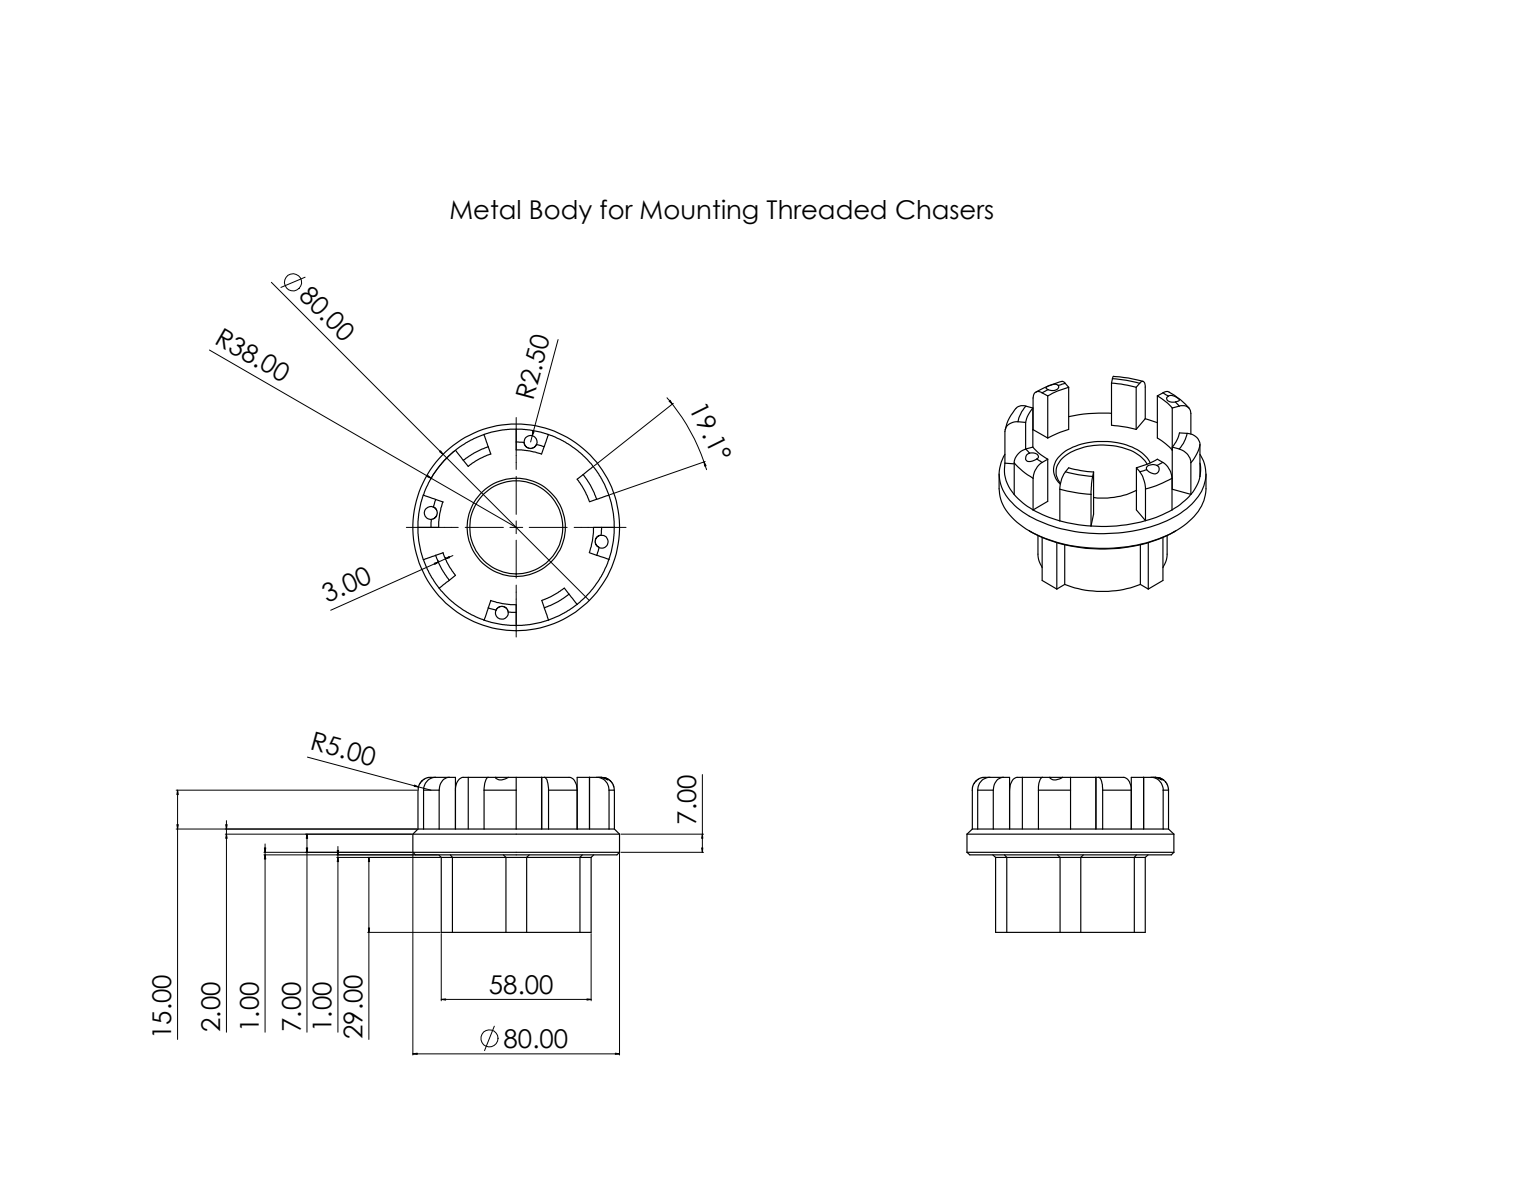
ISO-10303-21;
HEADER;
FILE_DESCRIPTION (('STEP AP214'),
    '1' );
FILE_NAME ('Metal Body for Mounting Threaded Chasers.step',
    '2026-10-19T14:05:14',
    ( '' ),
    ( '' ),
    'SwSTEP 2.0',
    'SolidWorks 2025',
    '' );
FILE_SCHEMA (( 'AUTOMOTIVE_DESIGN' ));
ENDSEC;

DATA;
#1=AXIS2_PLACEMENT_3D ( 'NONE', #3987, #6980, #243 ) ;
#2=CARTESIAN_POINT ( 'NONE',  ( -12.48950176432141923, 54.99999999999999289, -35.88888888888889284 ) ) ;
#16=CARTESIAN_POINT ( 'NONE',  ( 0.000000000000000000, 39.99999999999999289, 0.000000000000000000 ) ) ;
#17=ORIENTED_EDGE ( 'NONE', *, *, #1471, .T. ) ;
#22=VERTEX_POINT ( 'NONE', #2863 ) ;
#23=CARTESIAN_POINT ( 'NONE',  ( -7.995545880304240960, 59.98659813632739457, 32.45264704635820152 ) ) ;
#26=ORIENTED_EDGE ( 'NONE', *, *, #454, .F. ) ;
#28=AXIS2_PLACEMENT_3D ( 'NONE', #4537, #730, #2939 ) ;
#31=DIRECTION ( 'NONE',  ( 0.000000000000000000, 0.000000000000000000, 1.000000000000000000 ) ) ;
#33=CARTESIAN_POINT ( 'NONE',  ( 28.34870838944214100, 59.99999999999999289, 9.815840903884559765 ) ) ;
#39=VECTOR ( 'NONE', #8891, 1000.000000000000000 ) ;
#40=CARTESIAN_POINT ( 'NONE',  ( -8.673617379884032514E-16, 30.00000000000000000, -4.000000000000002665 ) ) ;
#48=ADVANCED_FACE ( 'NONE', ( #1481 ), #9105, .T. ) ;
#52=ORIENTED_EDGE ( 'NONE', *, *, #3525, .F. ) ;
#53=CARTESIAN_POINT ( 'NONE',  ( 38.00000000000000711, 59.99999999999999289, 1.288922537256478387E-13 ) ) ;
#59=DIRECTION ( 'NONE',  ( -1.000000000000000000, 0.000000000000000000, 1.084202172485503448E-16 ) ) ;
#60=ORIENTED_EDGE ( 'NONE', *, *, #1877, .F. ) ;
#61=AXIS2_PLACEMENT_3D ( 'NONE', #6025, #2270, #8317 ) ;
#63=PRODUCT_CONTEXT ( 'NONE', #3923, 'mechanical' ) ;
#68=CARTESIAN_POINT ( 'NONE',  ( -3.999999999999999112, 28.99999999999997158, 24.67792535850613334 ) ) ;
#69=ORIENTED_EDGE ( 'NONE', *, *, #3277, .T. ) ;
#71=VERTEX_POINT ( 'NONE', #9199 ) ;
#73=DIRECTION ( 'NONE',  ( 0.000000000000000000, 1.000000000000000000, 0.000000000000000000 ) ) ;
#74=EDGE_CURVE ( 'NONE', #2204, #4788, #7083, .T. ) ;
#78=CARTESIAN_POINT ( 'NONE',  ( 28.33333333333337478, 39.99999999999999289, -9.860132971832594961 ) ) ;
#79=CARTESIAN_POINT ( 'NONE',  ( 20.99999999999999645, 30.00000000000000000, 4.000000000000000888 ) ) ;
#86=DIRECTION ( 'NONE',  ( 0.000000000000000000, 0.000000000000000000, 1.000000000000000000 ) ) ;
#91=ORIENTED_EDGE ( 'NONE', *, *, #7636, .T. ) ;
#92=CARTESIAN_POINT ( 'NONE',  ( 5.562309845534588959, 49.99999999999999289, -33.06426808735054124 ) ) ;
#95=CARTESIAN_POINT ( 'NONE',  ( 24.67792535850613334, 0.000000000000000000, 4.000000000000000888 ) ) ;
#96=CARTESIAN_POINT ( 'NONE',  ( 0.000000000000000000, 0.000000000000000000, 0.000000000000000000 ) ) ;
#99=DIRECTION ( 'NONE',  ( 0.9449569463147374782, 0.000000000000000000, 0.3271946967961527619 ) ) ;
#101=DIRECTION ( 'NONE',  ( 0.000000000000000000, -1.000000000000000000, 0.000000000000000000 ) ) ;
#105=AXIS2_PLACEMENT_3D ( 'NONE', #139, #1748, #4771 ) ;
#106=EDGE_CURVE ( 'NONE', #1933, #8061, #806, .T. ) ;
#108=VECTOR ( 'NONE', #4796, 1000.000000000000000 ) ;
#115=ADVANCED_FACE ( 'NONE', ( #5243 ), #6016, .F. ) ;
#120=CLOSED_SHELL ( 'NONE', ( #1419, #7952, #2099, #3958, #3679, #8907, #3700, #3725, #1256, #288, #9736, #7646, #7332, #6776, #8180, #48, #7507, #2171, #4864, #7401, #2702, #2733, #7456, #636, #936, #1118, #6024, #1058, #540, #1404, #1588, #7209, #115, #1059, #588, #939, #8009, #6508, #1237, #2007, #4157, #6912, #2948, #702, #4090, #7822, #4876, #3409, #2741, #2560, #1004, #4751, #8856, #1093, #818, #5216, #1926, #9214, #9112, #7707, #4600, #634, #1660, #1234, #9684, #1433, #2142, #7068, #5305, #2300, #8588, #5110, #8978, #5514, #6739, #8244, #7533, #7708, #9094, #6502, #6348, #7871, #6449, #6840, #9282, #4029, #5531, #4774, #891, #5599, #3099, #5594, #5412, #1186, #7274, #6763, #3544, #3838, #1663, #3596, #7633, #5416, #9580, #6826, #5045, #4533, #1363 ) ) ;
#121=ORIENTED_EDGE ( 'NONE', *, *, #2139, .T. ) ;
#123=ORIENTED_EDGE ( 'NONE', *, *, #454, .T. ) ;
#127=LINE ( 'NONE', #9051, #3388 ) ;
#130=ORIENTED_EDGE ( 'NONE', *, *, #5654, .T. ) ;
#132=CARTESIAN_POINT ( 'NONE',  ( 4.000000000000001776, 28.99999999999997158, -24.67792535850613334 ) ) ;
#135=DIRECTION ( 'NONE',  ( -0.000000000000000000, -1.000000000000000000, -0.000000000000000000 ) ) ;
#137=VERTEX_POINT ( 'NONE', #6145 ) ;
#139=CARTESIAN_POINT ( 'NONE',  ( 0.000000000000000000, 54.99999999999999289, 0.000000000000000000 ) ) ;
#140=CARTESIAN_POINT ( 'NONE',  ( 32.85680095556730862, 59.99999999999999289, 3.070933240276029874 ) ) ;
#141=ORIENTED_EDGE ( 'NONE', *, *, #4576, .F. ) ;
#142=DIRECTION ( 'NONE',  ( -0.000000000000000000, -1.000000000000000000, -0.000000000000000000 ) ) ;
#143=ORIENTED_EDGE ( 'NONE', *, *, #5654, .F. ) ;
#151=CARTESIAN_POINT ( 'NONE',  ( 4.000000000000007994, 30.00000000000000000, 24.67792535850613334 ) ) ;
#152=CARTESIAN_POINT ( 'NONE',  ( 5.562309845534588959, 59.99999999999999289, -30.56426808735054479 ) ) ;
#156=VERTEX_POINT ( 'NONE', #6690 ) ;
#165=CARTESIAN_POINT ( 'NONE',  ( -4.331874290630486790, 29.33187429063046991, 24.96033808169876878 ) ) ;
#167=VERTEX_POINT ( 'NONE', #7496 ) ;
#174=CARTESIAN_POINT ( 'NONE',  ( 4.000000000000002665, 30.00000000000000000, -8.673617379884032514E-16 ) ) ;
#177=ORIENTED_EDGE ( 'NONE', *, *, #6292, .F. ) ;
#178=CARTESIAN_POINT ( 'NONE',  ( -7.935670091272695181, 60.00000000000000711, 32.24976038726180860 ) ) ;
#179=VERTEX_POINT ( 'NONE', #3191 ) ;
#183=CIRCLE ( 'NONE', #5688, 37.99999999999999289 ) ;
#186=CARTESIAN_POINT ( 'NONE',  ( -29.00000000000000355, 30.00000000000000000, 4.000000000000010658 ) ) ;
#187=LINE ( 'NONE', #9125, #4256 ) ;
#190=DIRECTION ( 'NONE',  ( 0.000000000000000000, -0.000000000000000000, 1.000000000000000000 ) ) ;
#191=CARTESIAN_POINT ( 'NONE',  ( 7.856683717344210116, 59.59863544270934455, -34.07748394475226661 ) ) ;
#192=LINE ( 'NONE', #2440, #6007 ) ;
#194=CARTESIAN_POINT ( 'NONE',  ( 0.000000000000000000, 54.99999999999999289, 0.000000000000000000 ) ) ;
#196=CARTESIAN_POINT ( 'NONE',  ( 12.43339847825378364, 39.99999999999999289, -35.90836395996003461 ) ) ;
#201=EDGE_CURVE ( 'NONE', #5205, #8953, #1759, .T. ) ;
#204=CARTESIAN_POINT ( 'NONE',  ( 33.06426808735054124, 59.99576382555915899, 3.062309845534584074 ) ) ;
#206=AXIS2_PLACEMENT_3D ( 'NONE', #7812, #2466, #1194 ) ;
#207=CARTESIAN_POINT ( 'NONE',  ( 0.000000000000000000, 30.00000000000000000, 0.000000000000000000 ) ) ;
#208=DIRECTION ( 'NONE',  ( 0.000000000000000000, -1.000000000000000000, 0.000000000000000000 ) ) ;
#209=VERTEX_POINT ( 'NONE', #7698 ) ;
#215=ORIENTED_EDGE ( 'NONE', *, *, #2320, .T. ) ;
#218=ORIENTED_EDGE ( 'NONE', *, *, #4973, .T. ) ;
#219=CARTESIAN_POINT ( 'NONE',  ( 33.06426808735054124, 49.99999999999999289, 5.562309845534586294 ) ) ;
#220=AXIS2_PLACEMENT_3D ( 'NONE', #9694, #2922, #5107 ) ;
#223=EDGE_CURVE ( 'NONE', #5194, #1935, #3139, .T. ) ;
#227=ORIENTED_EDGE ( 'NONE', *, *, #8008, .F. ) ;
#228=CARTESIAN_POINT ( 'NONE',  ( -33.72085295419949347, 59.72647237447257851, -7.995677060003914427 ) ) ;
#230=ORIENTED_EDGE ( 'NONE', *, *, #1372, .F. ) ;
#231=ORIENTED_EDGE ( 'NONE', *, *, #8364, .T. ) ;
#234=FACE_OUTER_BOUND ( 'NONE', #8971, .T. ) ;
#236=ORIENTED_EDGE ( 'NONE', *, *, #3146, .F. ) ;
#237=EDGE_CURVE ( 'NONE', #1437, #3718, #3681, .T. ) ;
#238=ORIENTED_EDGE ( 'NONE', *, *, #9403, .F. ) ;
#243=DIRECTION ( 'NONE',  ( 0.000000000000000000, 0.000000000000000000, 1.000000000000000000 ) ) ;
#247=ORIENTED_EDGE ( 'NONE', *, *, #9110, .F. ) ;
#252=VERTEX_POINT ( 'NONE', #7632 ) ;
#264=VECTOR ( 'NONE', #8760, 1000.000000000000000 ) ;
#267=CARTESIAN_POINT ( 'NONE',  ( 0.000000000000000000, 37.99999999999996447, -40.00000000000000711 ) ) ;
#268=PLANE ( 'NONE',  #1365 ) ;
#270=AXIS2_PLACEMENT_3D ( 'NONE', #2075, #7132, #3665 ) ;
#275=ORIENTED_EDGE ( 'NONE', *, *, #6897, .F. ) ;
#276=CARTESIAN_POINT ( 'NONE',  ( -35.47893788052810038, 58.98370868798952671, -6.231324730575372506 ) ) ;
#279=VERTEX_POINT ( 'NONE', #6422 ) ;
#280=EDGE_CURVE ( 'NONE', #8145, #2204, #7893, .T. ) ;
#287=CARTESIAN_POINT ( 'NONE',  ( 3.060768115627997776, 59.99034304420147379, -33.21665709534246957 ) ) ;
#288=ADVANCED_FACE ( 'NONE', ( #6098 ), #6191, .T. ) ;
#289=PLANE ( 'NONE',  #8040 ) ;
#290=EDGE_CURVE ( 'NONE', #22, #2244, #187, .T. ) ;
#291=CARTESIAN_POINT ( 'NONE',  ( 33.00000000000000711, 59.99999999999999289, 1.152188841818234386E-13 ) ) ;
#294=VERTEX_POINT ( 'NONE', #8424 ) ;
#295=CARTESIAN_POINT ( 'NONE',  ( -2.653525817520781855E-13, 39.99999999999999289, 38.00000000000000711 ) ) ;
#300=VERTEX_POINT ( 'NONE', #423 ) ;
#303=CARTESIAN_POINT ( 'NONE',  ( 0.000000000000000000, 28.99999999999997158, 0.000000000000000000 ) ) ;
#307=LINE ( 'NONE', #9387, #9703 ) ;
#308=ORIENTED_EDGE ( 'NONE', *, *, #4770, .F. ) ;
#310=ORIENTED_EDGE ( 'NONE', *, *, #635, .T. ) ;
#311=VECTOR ( 'NONE', #5751, 1000.000000000000000 ) ;
#312=DIRECTION ( 'NONE',  ( 0.000000000000000000, 1.000000000000000000, 0.000000000000000000 ) ) ;
#313=CARTESIAN_POINT ( 'NONE',  ( -5.562309845534584518, 49.99999999999999289, 35.56426808735054834 ) ) ;
#314=ORIENTED_EDGE ( 'NONE', *, *, #2672, .F. ) ;
#316=ORIENTED_EDGE ( 'NONE', *, *, #2562, .T. ) ;
#317=CARTESIAN_POINT ( 'NONE',  ( 0.000000000000000000, 1.000000000000014655, 0.000000000000000000 ) ) ;
#323=CARTESIAN_POINT ( 'NONE',  ( 23.54469556655648077, 59.99999999999999289, 29.82695610816123022 ) ) ;
#325=CIRCLE ( 'NONE', #6298, 38.00000000000000711 ) ;
#327=CARTESIAN_POINT ( 'NONE',  ( 2.326828918379978070E-15, 39.99999999999999289, -19.00000000000005684 ) ) ;
#330=DIRECTION ( 'NONE',  ( -0.9444444444444315412, 0.000000000000000000, 0.3286710990611268479 ) ) ;
#333=AXIS2_PLACEMENT_3D ( 'NONE', #8336, #1619, #1570 ) ;
#334=CARTESIAN_POINT ( 'NONE',  ( 33.06426808735054124, 49.99999999999999289, 3.062309845534584074 ) ) ;
#337=EDGE_CURVE ( 'NONE', #8698, #5898, #9303, .T. ) ;
#338=EDGE_LOOP ( 'NONE', ( #2836, #3852, #9165, #3920 ) ) ;
#339=CARTESIAN_POINT ( 'NONE',  ( -27.66666666666669272, 27.66666666666662167, 2.666666666666698049 ) ) ;
#342=DIRECTION ( 'NONE',  ( 0.000000000000000000, 0.000000000000000000, 1.000000000000000000 ) ) ;
#343=CARTESIAN_POINT ( 'NONE',  ( 0.000000000000000000, 0.000000000000000000, -19.00000000000000355 ) ) ;
#352=EDGE_CURVE ( 'NONE', #8330, #6149, #3299, .T. ) ;
#354=EDGE_LOOP ( 'NONE', ( #1511, #1589, #3120, #2364 ) ) ;
#355=DIRECTION ( 'NONE',  ( 0.000000000000000000, 0.000000000000000000, 1.000000000000000000 ) ) ;
#360=LINE ( 'NONE', #5642, #2706 ) ;
#361=CYLINDRICAL_SURFACE ( 'NONE', #4515, 2.500000000000002220 ) ;
#365=CARTESIAN_POINT ( 'NONE',  ( 4.000000000000001776, 28.99999999999997158, -29.00000000000000355 ) ) ;
#367=ORIENTED_EDGE ( 'NONE', *, *, #5413, .T. ) ;
#370=ORIENTED_EDGE ( 'NONE', *, *, #6332, .F. ) ;
#374=VECTOR ( 'NONE', #842, 1000.000000000000000 ) ;
#378=CARTESIAN_POINT ( 'NONE',  ( 29.00000000000000355, 0.000000000000000000, 4.000000000000000000 ) ) ;
#380=PLANE ( 'NONE',  #9644 ) ;
#381=LINE ( 'NONE', #8854, #6240 ) ;
#384=LINE ( 'NONE', #5665, #2838 ) ;
#389=CARTESIAN_POINT ( 'NONE',  ( 29.00000000000000355, 28.99999999999997158, 4.000000000000000000 ) ) ;
#394=ORIENTED_EDGE ( 'NONE', *, *, #7055, .T. ) ;
#396=EDGE_CURVE ( 'NONE', #1074, #9346, #9245, .T. ) ;
#397=CARTESIAN_POINT ( 'NONE',  ( -9.860132971832692661, 59.99999999999999289, -28.33333333333334281 ) ) ;
#401=DIRECTION ( 'NONE',  ( 0.000000000000000000, 0.000000000000000000, -1.000000000000000000 ) ) ;
#403=CARTESIAN_POINT ( 'NONE',  ( -25.51470164434615029, 30.00000000000000000, 5.000000000000010658 ) ) ;
#404=VECTOR ( 'NONE', #5914, 1000.000000000000000 ) ;
#405=CIRCLE ( 'NONE', #6383, 25.00000000000000000 ) ;
#406=ORIENTED_EDGE ( 'NONE', *, *, #5172, .F. ) ;
#407=CARTESIAN_POINT ( 'NONE',  ( 32.89361530837994962, 59.92713194881500982, 8.062309845534587183 ) ) ;
#410=ORIENTED_EDGE ( 'NONE', *, *, #3584, .F. ) ;
#413=CARTESIAN_POINT ( 'NONE',  ( -9.860132971832692661, 39.99999999999999289, -28.33333333333334281 ) ) ;
#418=AXIS2_PLACEMENT_3D ( 'NONE', #5812, #3538, #4432 ) ;
#423=CARTESIAN_POINT ( 'NONE',  ( -3.999999999999998224, 0.000000000000000000, 29.00000000000000355 ) ) ;
#427=VERTEX_POINT ( 'NONE', #5125 ) ;
#428=DIRECTION ( 'NONE',  ( 0.000000000000000000, 0.000000000000000000, 1.000000000000000000 ) ) ;
#430=ORIENTED_EDGE ( 'NONE', *, *, #1372, .T. ) ;
#437=ORIENTED_EDGE ( 'NONE', *, *, #7689, .F. ) ;
#438=FACE_OUTER_BOUND ( 'NONE', #6312, .T. ) ;
#439=FACE_OUTER_BOUND ( 'NONE', #470, .T. ) ;
#441=DIRECTION ( 'NONE',  ( 0.000000000000000000, 0.000000000000000000, 1.000000000000000000 ) ) ;
#446=ORIENTED_EDGE ( 'NONE', *, *, #6627, .T. ) ;
#448=DIRECTION ( 'NONE',  ( 0.000000000000000000, 0.7071067811865474617, 0.7071067811865474617 ) ) ;
#450=DIRECTION ( 'NONE',  ( 0.000000000000000000, 0.000000000000000000, 1.000000000000000000 ) ) ;
#452=DIRECTION ( 'NONE',  ( 0.7071067811865573427, -0.7071067811865376918, -0.000000000000000000 ) ) ;
#454=EDGE_CURVE ( 'NONE', #4849, #1467, #8923, .T. ) ;
#460=DIRECTION ( 'NONE',  ( 0.6195972517514876099, -0.000000000000000000, 0.7849198975831889191 ) ) ;
#470=EDGE_LOOP ( 'NONE', ( #5916, #4580, #3218, #2134, #8926 ) ) ;
#471=DIRECTION ( 'NONE',  ( 0.9444444444444359821, 0.000000000000000000, -0.3286710990611142469 ) ) ;
#472=EDGE_LOOP ( 'NONE', ( #7982, #7930, #8063, #3856 ) ) ;
#475=DIRECTION ( 'NONE',  ( -0.000000000000000000, -1.000000000000000000, -0.000000000000000000 ) ) ;
#479=DIRECTION ( 'NONE',  ( 0.000000000000000000, 0.000000000000000000, 1.000000000000000000 ) ) ;
#489=ORIENTED_EDGE ( 'NONE', *, *, #3270, .T. ) ;
#494=EDGE_LOOP ( 'NONE', ( #6497, #4079, #9500, #4446, #1743, #1658, #5716 ) ) ;
#504=VERTEX_POINT ( 'NONE', #5174 ) ;
#509=EDGE_CURVE ( 'NONE', #4792, #7168, #1410, .T. ) ;
#511=CIRCLE ( 'NONE', #8869, 5.000000000000001776 ) ;
#514=CARTESIAN_POINT ( 'NONE',  ( 0.000000000000000000, 30.00000000000000000, 0.000000000000000000 ) ) ;
#516=CARTESIAN_POINT ( 'NONE',  ( -4.000000000000005329, 28.99999999999997158, -29.00000000000000355 ) ) ;
#522=DIRECTION ( 'NONE',  ( -0.7849198975831889191, -0.000000000000000000, 0.6195972517514874989 ) ) ;
#527=ORIENTED_EDGE ( 'NONE', *, *, #2371, .T. ) ;
#529=CARTESIAN_POINT ( 'NONE',  ( 28.33333333333337833, 59.99999999999999289, -9.860132971832594961 ) ) ;
#531=CARTESIAN_POINT ( 'NONE',  ( 4.000000000000001776, 0.000000000000000000, 0.000000000000000000 ) ) ;
#533=VECTOR ( 'NONE', #5958, 1000.000000000000000 ) ;
#535=EDGE_CURVE ( 'NONE', #4621, #5147, #2943, .T. ) ;
#538=EDGE_CURVE ( 'NONE', #6765, #4792, #5901, .T. ) ;
#540=ADVANCED_FACE ( 'NONE', ( #4241, #5074 ), #1370, .F. ) ;
#542=AXIS2_PLACEMENT_3D ( 'NONE', #8748, #5544, #7870 ) ;
#547=FACE_OUTER_BOUND ( 'NONE', #7373, .T. ) ;
#551=SHAPE_REPRESENTATION ( 'Metal Body for Mounting Threaded Chasers', ( #6314 ), #2843 ) ;
#555=DIRECTION ( 'NONE',  ( -0.000000000000000000, -1.000000000000000000, -0.000000000000000000 ) ) ;
#557=ORIENTED_EDGE ( 'NONE', *, *, #2320, .F. ) ;
#558=DIRECTION ( 'NONE',  ( -0.000000000000000000, -1.000000000000000000, -0.000000000000000000 ) ) ;
#563=CARTESIAN_POINT ( 'NONE',  ( -34.19425402209839859, 59.81545713833158828, -3.326151553796970806 ) ) ;
#564=ORIENTED_EDGE ( 'NONE', *, *, #4438, .T. ) ;
#565=CARTESIAN_POINT ( 'NONE',  ( 33.72911585420148128, 59.92558239856793278, 3.146586008005429314 ) ) ;
#566=ORIENTED_EDGE ( 'NONE', *, *, #352, .T. ) ;
#568=ORIENTED_EDGE ( 'NONE', *, *, #7347, .T. ) ;
#573=AXIS2_PLACEMENT_3D ( 'NONE', #9355, #2572, #5602 ) ;
#575=DIRECTION ( 'NONE',  ( 0.000000000000000000, -0.7071067811865500152, -0.7071067811865451302 ) ) ;
#579=ORIENTED_EDGE ( 'NONE', *, *, #6665, .T. ) ;
#585=CARTESIAN_POINT ( 'NONE',  ( 4.331874290630496560, 29.33187429063046991, 24.96033808169876878 ) ) ;
#588=ADVANCED_FACE ( 'NONE', ( #8138 ), #2885, .T. ) ;
#590=DIRECTION ( 'NONE',  ( -1.000000000000000000, 0.000000000000000000, 2.168404344971006649E-16 ) ) ;
#592=EDGE_CURVE ( 'NONE', #7004, #2792, #2691, .T. ) ;
#593=ORIENTED_EDGE ( 'NONE', *, *, #4388, .T. ) ;
#595=DIRECTION ( 'NONE',  ( 0.000000000000000000, 1.000000000000000000, 0.000000000000000000 ) ) ;
#596=DIRECTION ( 'NONE',  ( -0.000000000000000000, -1.000000000000000000, -0.000000000000000000 ) ) ;
#598=ORIENTED_EDGE ( 'NONE', *, *, #5533, .T. ) ;
#602=CARTESIAN_POINT ( 'NONE',  ( -9.860132971832692661, 59.99999999999999289, -28.33333333333334281 ) ) ;
#604=EDGE_LOOP ( 'NONE', ( #4455, #8847, #6470, #2076 ) ) ;
#609=ORIENTED_EDGE ( 'NONE', *, *, #1964, .F. ) ;
#619=ORIENTED_EDGE ( 'NONE', *, *, #8790, .F. ) ;
#620=FACE_OUTER_BOUND ( 'NONE', #3521, .T. ) ;
#621=DIRECTION ( 'NONE',  ( 0.000000000000000000, -1.000000000000000000, 0.000000000000000000 ) ) ;
#622=DIRECTION ( 'NONE',  ( 0.000000000000000000, 0.000000000000000000, 1.000000000000000000 ) ) ;
#623=DIRECTION ( 'NONE',  ( 0.3271946967961529840, 0.000000000000000000, -0.9449569463147373671 ) ) ;
#624=DIRECTION ( 'NONE',  ( -0.000000000000000000, -1.000000000000000000, -0.000000000000000000 ) ) ;
#634=ADVANCED_FACE ( 'NONE', ( #4391 ), #5023, .F. ) ;
#635=EDGE_CURVE ( 'NONE', #5898, #2818, #5499, .T. ) ;
#636=ADVANCED_FACE ( 'NONE', ( #9571 ), #1321, .T. ) ;
#645=AXIS2_PLACEMENT_3D ( 'NONE', #194, #4729, #6198 ) ;
#654=ORIENTED_EDGE ( 'NONE', *, *, #4759, .F. ) ;
#655=DIRECTION ( 'NONE',  ( 0.000000000000000000, 0.000000000000000000, 1.000000000000000000 ) ) ;
#657=CARTESIAN_POINT ( 'NONE',  ( 35.48172963891341425, 59.13032414405947179, 4.904055200121585578 ) ) ;
#662=DIRECTION ( 'NONE',  ( 0.000000000000000000, 1.000000000000000000, 0.000000000000000000 ) ) ;
#666=ORIENTED_EDGE ( 'NONE', *, *, #2923, .F. ) ;
#674=CARTESIAN_POINT ( 'NONE',  ( 0.000000000000000000, 54.99999999999999289, 0.000000000000000000 ) ) ;
#685=B_SPLINE_CURVE_WITH_KNOTS ( 'NONE', 3,
 ( #9148, #1636, #3056, #5346 ),
 .UNSPECIFIED., .F., .F.,
 ( 4, 4 ),
 ( 0.000000000000000000, 0.001643226871903046308 ),
 .UNSPECIFIED. ) ;
#687=CARTESIAN_POINT ( 'NONE',  ( 20.99999999999999645, 30.00000000000000000, -4.000000000000006217 ) ) ;
#688=EDGE_LOOP ( 'NONE', ( #2555, #5795, #446, #121 ) ) ;
#690=EDGE_CURVE ( 'NONE', #5689, #4621, #1513, .T. ) ;
#691=ORIENTED_EDGE ( 'NONE', *, *, #2255, .T. ) ;
#697=LINE ( 'NONE', #6703, #2761 ) ;
#702=ADVANCED_FACE ( 'NONE', ( #881 ), #5993, .F. ) ;
#704=CARTESIAN_POINT ( 'NONE',  ( 35.54672840350796292, 58.97502204235875922, 5.902312647278757929 ) ) ;
#711=EDGE_LOOP ( 'NONE', ( #4221, #2161, #4934, #4957, #6130 ) ) ;
#712=DIRECTION ( 'NONE',  ( -0.000000000000000000, -1.000000000000000000, -0.000000000000000000 ) ) ;
#715=VECTOR ( 'NONE', #596, 1000.000000000000000 ) ;
#716=ORIENTED_EDGE ( 'NONE', *, *, #8054, .F. ) ;
#717=DIRECTION ( 'NONE',  ( 0.000000000000000000, 0.000000000000000000, -1.000000000000000000 ) ) ;
#720=DIRECTION ( 'NONE',  ( 0.000000000000000000, 0.000000000000000000, -1.000000000000000000 ) ) ;
#722=DIRECTION ( 'NONE',  ( 0.000000000000000000, 0.000000000000000000, -1.000000000000000000 ) ) ;
#723=( NAMED_UNIT ( * ) PLANE_ANGLE_UNIT ( ) SI_UNIT ( $, .RADIAN. ) );
#725=VECTOR ( 'NONE', #4013, 1000.000000000000000 ) ;
#726=AXIS2_PLACEMENT_3D ( 'NONE', #2931, #8863, #5748 ) ;
#730=DIRECTION ( 'NONE',  ( -1.000000000000000000, 0.000000000000000000, -6.982962677686269077E-15 ) ) ;
#734=CARTESIAN_POINT ( 'NONE',  ( -5.000000000000002665, 30.00000000000000000, 5.421010862427519212E-16 ) ) ;
#736=CIRCLE ( 'NONE', #5785, 40.00000000000000711 ) ;
#739=ORIENTED_EDGE ( 'NONE', *, *, #3429, .F. ) ;
#742=VERTEX_POINT ( 'NONE', #2390 ) ;
#744=AXIS2_PLACEMENT_3D ( 'NONE', #8928, #8876, #3589 ) ;
#745=CARTESIAN_POINT ( 'NONE',  ( -5.421010862427522170E-16, 30.00000000000000000, -5.000000000000004441 ) ) ;
#754=ORIENTED_EDGE ( 'NONE', *, *, #2562, .F. ) ;
#757=CARTESIAN_POINT ( 'NONE',  ( 0.000000000000000000, 54.99999999999999289, 0.000000000000000000 ) ) ;
#758=DIRECTION ( 'NONE',  ( -0.7071067811865573427, 0.7071067811865376918, 0.000000000000000000 ) ) ;
#759=CARTESIAN_POINT ( 'NONE',  ( 23.54759692749571087, 59.99999999999999289, -18.58791755254458167 ) ) ;
#764=CARTESIAN_POINT ( 'NONE',  ( 32.99503133754566875, 59.99860354191589806, 3.062309845534584074 ) ) ;
#768=FACE_OUTER_BOUND ( 'NONE', #8392, .T. ) ;
#774=EDGE_LOOP ( 'NONE', ( #566, #4057 ) ) ;
#780=LINE ( 'NONE', #7737, #4904 ) ;
#783=AXIS2_PLACEMENT_3D ( 'NONE', #4118, #4582, #7112 ) ;
#784=CIRCLE ( 'NONE', #5829, 33.00000000000000711 ) ;
#788=CARTESIAN_POINT ( 'NONE',  ( -5.562309845534584518, 49.99999999999999289, 35.56426808735054834 ) ) ;
#790=EDGE_CURVE ( 'NONE', #2152, #2914, #4725, .T. ) ;
#794=AXIS2_PLACEMENT_3D ( 'NONE', #33, #7686, #6097 ) ;
#801=EDGE_LOOP ( 'NONE', ( #7375, #4405, #5867, #3569 ) ) ;
#806=B_SPLINE_CURVE_WITH_KNOTS ( 'NONE', 3,
 ( #9050, #9248, #6810, #1591 ),
 .UNSPECIFIED., .F., .F.,
 ( 4, 4 ),
 ( 0.000000000000000000, 0.001643226871903047392 ),
 .UNSPECIFIED. ) ;
#809=AXIS2_PLACEMENT_3D ( 'NONE', #3438, #7888, #1997 ) ;
#810=EDGE_CURVE ( 'NONE', #7824, #1842, #4038, .T. ) ;
#812=CARTESIAN_POINT ( 'NONE',  ( -5.775154784098236682, 58.97791112757357723, 35.56426808734908462 ) ) ;
#815=EDGE_LOOP ( 'NONE', ( #247, #8601, #275, #4670 ) ) ;
#818=ADVANCED_FACE ( 'NONE', ( #7842 ), #380, .T. ) ;
#819=DIRECTION ( 'NONE',  ( -0.000000000000000000, -1.000000000000000000, -0.000000000000000000 ) ) ;
#820=CARTESIAN_POINT ( 'NONE',  ( 5.562309845551833831, 59.00253480853272947, -35.56426808735054834 ) ) ;
#826=ORIENTED_EDGE ( 'NONE', *, *, #1722, .F. ) ;
#827=CARTESIAN_POINT ( 'NONE',  ( 2.204364238465235033E-15, -50.91168824543140659, -17.99999999999999645 ) ) ;
#828=AXIS2_PLACEMENT_3D ( 'NONE', #5685, #4218, #5543 ) ;
#831=EDGE_CURVE ( 'NONE', #6918, #8994, #969, .T. ) ;
#832=DIRECTION ( 'NONE',  ( -0.000000000000000000, 1.000000000000000000, -0.000000000000000000 ) ) ;
#834=EDGE_CURVE ( 'NONE', #4792, #6355, #8574, .T. ) ;
#835=LINE ( 'NONE', #3841, #4426 ) ;
#836=ORIENTED_EDGE ( 'NONE', *, *, #6420, .T. ) ;
#839=EDGE_LOOP ( 'NONE', ( #6390, #5258, #3782, #4715, #3267 ) ) ;
#840=FACE_OUTER_BOUND ( 'NONE', #8194, .T. ) ;
#841=EDGE_LOOP ( 'NONE', ( #4909, #7923, #1571, #5597 ) ) ;
#842=DIRECTION ( 'NONE',  ( -0.000000000000000000, 1.000000000000000000, -0.000000000000000000 ) ) ;
#844=AXIS2_PLACEMENT_3D ( 'NONE', #1890, #1990, #1847 ) ;
#847=CARTESIAN_POINT ( 'NONE',  ( -30.00000000000000711, 30.00000000000000000, 5.000000000000011546 ) ) ;
#858=ORIENTED_EDGE ( 'NONE', *, *, #834, .F. ) ;
#862=VECTOR ( 'NONE', #2490, 1000.000000000000000 ) ;
#863=ORIENTED_EDGE ( 'NONE', *, *, #1217, .F. ) ;
#864=CARTESIAN_POINT ( 'NONE',  ( 32.85680095556730862, 59.99999999999999289, 3.070933240276029874 ) ) ;
#865=ORIENTED_EDGE ( 'NONE', *, *, #1471, .F. ) ;
#870=AXIS2_PLACEMENT_3D ( 'NONE', #3899, #2299, #4731 ) ;
#871=AXIS2_PLACEMENT_3D ( 'NONE', #7357, #8885, #5724 ) ;
#872=FACE_OUTER_BOUND ( 'NONE', #7624, .T. ) ;
#876=DIRECTION ( 'NONE',  ( -0.3271946967961539277, 0.000000000000000000, 0.9449569463147370341 ) ) ;
#877=CIRCLE ( 'NONE', #6381, 33.00000000000000711 ) ;
#878=CARTESIAN_POINT ( 'NONE',  ( -3.516611797194481248, 59.70849920474193340, 34.51129295977867883 ) ) ;
#880=VERTEX_POINT ( 'NONE', #9420 ) ;
#881=FACE_OUTER_BOUND ( 'NONE', #3150, .T. ) ;
#885=ORIENTED_EDGE ( 'NONE', *, *, #5170, .T. ) ;
#887=VECTOR ( 'NONE', #9049, 1000.000000000000000 ) ;
#891=ADVANCED_FACE ( 'NONE', ( #8075 ), #3481, .F. ) ;
#893=VECTOR ( 'NONE', #2160, 1000.000000000000000 ) ;
#894=DIRECTION ( 'NONE',  ( 0.000000000000000000, 0.000000000000000000, 1.000000000000000000 ) ) ;
#899=DIRECTION ( 'NONE',  ( -1.000000000000000000, 0.000000000000000000, -1.047444401652940795E-14 ) ) ;
#900=VECTOR ( 'NONE', #3307, 1000.000000000000000 ) ;
#907=ORIENTED_EDGE ( 'NONE', *, *, #4031, .F. ) ;
#908=CARTESIAN_POINT ( 'NONE',  ( -28.34870838944214455, 59.99999999999999289, -9.815840903884556212 ) ) ;
#909=VERTEX_POINT ( 'NONE', #5892 ) ;
#910=DIRECTION ( 'NONE',  ( 0.000000000000000000, 0.000000000000000000, 1.000000000000000000 ) ) ;
#911=DIRECTION ( 'NONE',  ( 0.6195972517514870548, -0.000000000000000000, 0.7849198975831892522 ) ) ;
#912=ORIENTED_EDGE ( 'NONE', *, *, #1001, .T. ) ;
#919=CARTESIAN_POINT ( 'NONE',  ( 0.000000000000000000, 59.99999999999999289, -33.00000000000000711 ) ) ;
#920=EDGE_LOOP ( 'NONE', ( #8639, #3272, #4380, #5538 ) ) ;
#921=DIRECTION ( 'NONE',  ( -0.000000000000000000, -1.000000000000000000, -0.000000000000000000 ) ) ;
#924=CARTESIAN_POINT ( 'NONE',  ( 4.861949598180850707, 59.13521925290943670, -35.48792514263537612 ) ) ;
#927=CARTESIAN_POINT ( 'NONE',  ( 0.000000000000000000, 30.99999999999998579, 0.000000000000000000 ) ) ;
#936=ADVANCED_FACE ( 'NONE', ( #1944, #1219 ), #1896, .F. ) ;
#939=ADVANCED_FACE ( 'NONE', ( #1264 ), #9558, .T. ) ;
#942=VECTOR ( 'NONE', #6726, 1000.000000000000000 ) ;
#948=CARTESIAN_POINT ( 'NONE',  ( 30.00000000000000711, 30.00000000000000000, 5.000000000000000888 ) ) ;
#950=EDGE_CURVE ( 'NONE', #6089, #8994, #8820, .T. ) ;
#951=VECTOR ( 'NONE', #5557, 1000.000000000000000 ) ;
#953=CARTESIAN_POINT ( 'NONE',  ( 25.51470164434615029, 30.00000000000000000, -5.000000000000007105 ) ) ;
#958=ORIENTED_EDGE ( 'NONE', *, *, #592, .T. ) ;
#964=CARTESIAN_POINT ( 'NONE',  ( -33.06426808735054124, 49.99999999999999289, -5.562309845534581854 ) ) ;
#966=ORIENTED_EDGE ( 'NONE', *, *, #4720, .T. ) ;
#967=PLANE ( 'NONE',  #794 ) ;
#969=LINE ( 'NONE', #2437, #5435 ) ;
#970=CARTESIAN_POINT ( 'NONE',  ( 7.935670091272698734, 60.00000000000000711, -32.24976038726181571 ) ) ;
#971=FACE_OUTER_BOUND ( 'NONE', #4525, .T. ) ;
#977=AXIS2_PLACEMENT_3D ( 'NONE', #5178, #8186, #3741 ) ;
#979=ORIENTED_EDGE ( 'NONE', *, *, #1214, .T. ) ;
#982=VERTEX_POINT ( 'NONE', #3580 ) ;
#983=EDGE_CURVE ( 'NONE', #1128, #427, #7232, .T. ) ;
#984=AXIS2_PLACEMENT_3D ( 'NONE', #219, #6220, #2324 ) ;
#986=LINE ( 'NONE', #1768, #108 ) ;
#988=EDGE_CURVE ( 'NONE', #1527, #1864, #4967, .T. ) ;
#995=DIRECTION ( 'NONE',  ( 0.3286710990611269034, -0.000000000000000000, 0.9444444444444316522 ) ) ;
#998=VECTOR ( 'NONE', #911, 1000.000000000000114 ) ;
#999=CARTESIAN_POINT ( 'NONE',  ( -12.48950176432141923, 39.99999999999999289, -35.88888888888889284 ) ) ;
#1001=EDGE_CURVE ( 'NONE', #8160, #1864, #7383, .T. ) ;
#1003=CARTESIAN_POINT ( 'NONE',  ( -35.21620900558183820, 59.09151583898437821, -6.845072491844675255 ) ) ;
#1004=ADVANCED_FACE ( 'NONE', ( #620 ), #2038, .F. ) ;
#1006=CARTESIAN_POINT ( 'NONE',  ( 34.69710844949434403, 59.33700357310857498, 7.462191142828216606 ) ) ;
#1007=ORIENTED_EDGE ( 'NONE', *, *, #3223, .T. ) ;
#1010=CARTESIAN_POINT ( 'NONE',  ( 0.000000000000000000, 54.99999999999999289, 0.000000000000000000 ) ) ;
#1014=PLANE ( 'NONE',  #7423 ) ;
#1017=VERTEX_POINT ( 'NONE', #6505 ) ;
#1021=CIRCLE ( 'NONE', #1963, 33.00000000000000711 ) ;
#1023=VECTOR ( 'NONE', #3636, 1000.000000000000000 ) ;
#1024=DIRECTION ( 'NONE',  ( -0.000000000000000000, -1.000000000000000000, -0.000000000000000000 ) ) ;
#1026=STYLED_ITEM('',(#9771),#6272);
#1029=CARTESIAN_POINT ( 'NONE',  ( -33.06426808735054124, 49.99999999999999289, -5.562309845534581854 ) ) ;
#1030=CARTESIAN_POINT ( 'NONE',  ( 38.00000000000000711, 54.99999999999999289, 1.288922537256478387E-13 ) ) ;
#1036=CARTESIAN_POINT ( 'NONE',  ( 0.000000000000000000, 59.99999999999999289, 0.000000000000000000 ) ) ;
#1037=CIRCLE ( 'NONE', #7977, 40.00000000000000711 ) ;
#1042=DIRECTION ( 'NONE',  ( 0.3271946967961528174, -0.000000000000000000, -0.9449569463147374782 ) ) ;
#1045=FACE_OUTER_BOUND ( 'NONE', #4412, .T. ) ;
#1046=ORIENTED_EDGE ( 'NONE', *, *, #4987, .T. ) ;
#1047=CIRCLE ( 'NONE', #9404, 40.00000000000000711 ) ;
#1048=DIRECTION ( 'NONE',  ( 0.000000000000000000, 1.000000000000000000, 0.000000000000000000 ) ) ;
#1049=FACE_OUTER_BOUND ( 'NONE', #4097, .T. ) ;
#1054=CARTESIAN_POINT ( 'NONE',  ( 33.39503079668222085, 59.82426665968211665, 8.062309845534590735 ) ) ;
#1055=ORIENTED_EDGE ( 'NONE', *, *, #509, .T. ) ;
#1058=ADVANCED_FACE ( 'NONE', ( #5031 ), #7403, .T. ) ;
#1059=ADVANCED_FACE ( 'NONE', ( #5622 ), #1075, .F. ) ;
#1065=CARTESIAN_POINT ( 'NONE',  ( -3.106744199778896931, 59.95265069314689299, 33.56539760714087350 ) ) ;
#1066=EDGE_LOOP ( 'NONE', ( #230, #5982, #5408, #2955 ) ) ;
#1068=DIRECTION ( 'NONE',  ( 0.000000000000000000, 1.000000000000000000, 0.000000000000000000 ) ) ;
#1069=DIRECTION ( 'NONE',  ( -0.000000000000000000, -1.000000000000000000, -0.000000000000000000 ) ) ;
#1070=DIRECTION ( 'NONE',  ( 0.000000000000000000, 0.000000000000000000, -1.000000000000000000 ) ) ;
#1071=EDGE_CURVE ( 'NONE', #1104, #8562, #9429, .T. ) ;
#1074=VERTEX_POINT ( 'NONE', #6985 ) ;
#1075=PLANE ( 'NONE',  #4000 ) ;
#1079=DIRECTION ( 'NONE',  ( 0.000000000000000000, 0.000000000000000000, 1.000000000000000000 ) ) ;
#1080=CARTESIAN_POINT ( 'NONE',  ( -8.673617379884032514E-16, 0.000000000000000000, -4.000000000000002665 ) ) ;
#1083=CARTESIAN_POINT ( 'NONE',  ( 2.326828918379971365E-15, 0.000000000000000000, 19.00000000000000355 ) ) ;
#1088=EDGE_CURVE ( 'NONE', #7168, #7878, #5669, .T. ) ;
#1091=CARTESIAN_POINT ( 'NONE',  ( 0.000000000000000000, 30.99999999999998579, 0.000000000000000000 ) ) ;
#1093=ADVANCED_FACE ( 'NONE', ( #4837 ), #7852, .F. ) ;
#1094=FACE_OUTER_BOUND ( 'NONE', #2624, .T. ) ;
#1096=DIRECTION ( 'NONE',  ( -0.000000000000000000, -1.000000000000000000, -0.000000000000000000 ) ) ;
#1097=VERTEX_POINT ( 'NONE', #7089 ) ;
#1098=CARTESIAN_POINT ( 'NONE',  ( 0.000000000000000000, 30.00000000000000000, 0.000000000000000000 ) ) ;
#1100=DIRECTION ( 'NONE',  ( 0.000000000000000000, 1.000000000000000000, -0.000000000000000000 ) ) ;
#1104=VERTEX_POINT ( 'NONE', #389 ) ;
#1105=AXIS2_PLACEMENT_3D ( 'NONE', #7741, #6051, #3943 ) ;
#1109=DIRECTION ( 'NONE',  ( 0.000000000000000000, 0.000000000000000000, 1.000000000000000000 ) ) ;
#1110=B_SPLINE_CURVE_WITH_KNOTS ( 'NONE', 3,
 ( #2960, #3153, #3758, #6751 ),
 .UNSPECIFIED., .F., .F.,
 ( 4, 4 ),
 ( 0.000000000000000000, 0.001643226871903046308 ),
 .UNSPECIFIED. ) ;
#1111=AXIS2_PLACEMENT_3D ( 'NONE', #5469, #3177, #9220 ) ;
#1115=CARTESIAN_POINT ( 'NONE',  ( -3.070933240276028542, 59.99999999999999289, 32.85680095556730862 ) ) ;
#1118=ADVANCED_FACE ( 'NONE', ( #8265 ), #3822, .F. ) ;
#1124=EDGE_CURVE ( 'NONE', #2244, #300, #8320, .T. ) ;
#1125=CARTESIAN_POINT ( 'NONE',  ( 0.000000000000000000, 39.99999999999999289, 0.000000000000000000 ) ) ;
#1128=VERTEX_POINT ( 'NONE', #3703 ) ;
#1133=ORIENTED_EDGE ( 'NONE', *, *, #1233, .F. ) ;
#1135=DIRECTION ( 'NONE',  ( -0.000000000000000000, -1.000000000000000000, -0.000000000000000000 ) ) ;
#1142=CARTESIAN_POINT ( 'NONE',  ( 32.37987785958423359, 59.99097422714241645, 7.973032508609962932 ) ) ;
#1143=DIRECTION ( 'NONE',  ( -0.3286710990611269034, 0.000000000000000000, -0.9444444444444315412 ) ) ;
#1144=AXIS2_PLACEMENT_3D ( 'NONE', #2062, #3604, #5187 ) ;
#1149=AXIS2_PLACEMENT_3D ( 'NONE', #9329, #4885, #1915 ) ;
#1151=ORIENTED_EDGE ( 'NONE', *, *, #2796, .T. ) ;
#1152=CARTESIAN_POINT ( 'NONE',  ( -33.39503079668222085, 59.82426665968211665, -8.062309845534588959 ) ) ;
#1160=CYLINDRICAL_SURFACE ( 'NONE', #7665, 30.00000000000000711 ) ;
#1165=CARTESIAN_POINT ( 'NONE',  ( 0.000000000000000000, 0.000000000000000000, 0.000000000000000000 ) ) ;
#1166=B_SPLINE_CURVE_WITH_KNOTS ( 'NONE', 3,
 ( #2835, #6543, #2982, #4479 ),
 .UNSPECIFIED., .F., .F.,
 ( 4, 4 ),
 ( 0.000000000000000000, 0.001643226871903046308 ),
 .UNSPECIFIED. ) ;
#1172=VECTOR ( 'NONE', #4829, 999.9999999999998863 ) ;
#1173=ORIENTED_EDGE ( 'NONE', *, *, #3240, .T. ) ;
#1176=ORIENTED_EDGE ( 'NONE', *, *, #7005, .T. ) ;
#1185=AXIS2_PLACEMENT_3D ( 'NONE', #2056, #2101, #2651 ) ;
#1186=ADVANCED_FACE ( 'NONE', ( #2768 ), #3846, .F. ) ;
#1187=CARTESIAN_POINT ( 'NONE',  ( 4.999999999999815259, 19.99999999999990763, 20.00000000000019185 ) ) ;
#1189=VECTOR ( 'NONE', #7916, 1000.000000000000000 ) ;
#1193=VERTEX_POINT ( 'NONE', #9320 ) ;
#1194=DIRECTION ( 'NONE',  ( 0.3271946967961539277, 0.000000000000000000, -0.9449569463147370341 ) ) ;
#1195=CONICAL_SURFACE ( 'NONE', #8930, 37.99999999999999289, 0.7853981633974447263 ) ;
#1196=AXIS2_PLACEMENT_3D ( 'NONE', #8264, #3118, #2972 ) ;
#1205=VECTOR ( 'NONE', #1593, 1000.000000000000000 ) ;
#1211=CARTESIAN_POINT ( 'NONE',  ( 0.000000000000000000, 59.99999999999999289, 0.000000000000000000 ) ) ;
#1213=AXIS2_PLACEMENT_3D ( 'NONE', #7796, #3345, #2493 ) ;
#1214=EDGE_CURVE ( 'NONE', #982, #6796, #5568, .T. ) ;
#1215=ORIENTED_EDGE ( 'NONE', *, *, #6641, .T. ) ;
#1217=EDGE_CURVE ( 'NONE', #6796, #4952, #9568, .T. ) ;
#1219=FACE_OUTER_BOUND ( 'NONE', #8915, .T. ) ;
#1222=DIRECTION ( 'NONE',  ( 0.000000000000000000, 1.000000000000000000, -0.000000000000000000 ) ) ;
#1223=DIRECTION ( 'NONE',  ( 0.000000000000000000, 0.000000000000000000, -1.000000000000000000 ) ) ;
#1226=CARTESIAN_POINT ( 'NONE',  ( -32.37987785958423359, 59.99097422714241645, -7.973032508609959379 ) ) ;
#1228=ORIENTED_EDGE ( 'NONE', *, *, #3352, .F. ) ;
#1233=EDGE_CURVE ( 'NONE', #7715, #4557, #1235, .T. ) ;
#1234=ADVANCED_FACE ( 'NONE', ( #439 ), #4182, .F. ) ;
#1235=B_SPLINE_CURVE_WITH_KNOTS ( 'NONE', 3,
 ( #5370, #7544, #2289, #3128, #3834, #8380, #3179, #3227, #878, #2388, #7029, #7840, #1065, #5701, #7230, #1115 ),
 .UNSPECIFIED., .F., .F.,
 ( 4, 2, 2, 2, 2, 2, 2, 4 ),
 ( 0.005084922178573568659, 0.006146119420698883951, 0.006676718041761538561, 0.007207316662824192303, 0.007737915283886846046, 0.008268513904949498922, 0.008799112526012153532, 0.009329711147074808142 ),
 .UNSPECIFIED. ) ;
#1237=ADVANCED_FACE ( 'NONE', ( #3328 ), #2678, .F. ) ;
#1246=EDGE_CURVE ( 'NONE', #4542, #9236, #5207, .T. ) ;
#1250=ORIENTED_EDGE ( 'NONE', *, *, #6050, .T. ) ;
#1251=CARTESIAN_POINT ( 'NONE',  ( 34.19425402209839859, 59.81545713833158828, 3.326151553796978355 ) ) ;
#1256=ADVANCED_FACE ( 'NONE', ( #3522 ), #7434, .T. ) ;
#1260=AXIS2_PLACEMENT_3D ( 'NONE', #2829, #4137, #4282 ) ;
#1261=ORIENTED_EDGE ( 'NONE', *, *, #7038, .F. ) ;
#1264=FACE_OUTER_BOUND ( 'NONE', #1066, .T. ) ;
#1265=DIRECTION ( 'NONE',  ( -1.047444401652940795E-14, -0.000000000000000000, 1.000000000000000000 ) ) ;
#1272=ORIENTED_EDGE ( 'NONE', *, *, #8570, .F. ) ;
#1277=DIRECTION ( 'NONE',  ( -0.000000000000000000, 1.000000000000000000, -0.000000000000000000 ) ) ;
#1279=FACE_OUTER_BOUND ( 'NONE', #2037, .T. ) ;
#1282=DIRECTION ( 'NONE',  ( -1.084202172485503448E-16, 0.000000000000000000, -1.000000000000000000 ) ) ;
#1283=DIRECTION ( 'NONE',  ( 0.000000000000000000, 0.000000000000000000, 1.000000000000000000 ) ) ;
#1284=VECTOR ( 'NONE', #7130, 1000.000000000000000 ) ;
#1285=ORIENTED_EDGE ( 'NONE', *, *, #4759, .T. ) ;
#1286=CYLINDRICAL_SURFACE ( 'NONE', #3506, 30.00000000000000711 ) ;
#1289=ORIENTED_EDGE ( 'NONE', *, *, #290, .F. ) ;
#1294=EDGE_LOOP ( 'NONE', ( #2608, #6117, #2414, #6412, #3983, #3371, #3119, #4801, #2703, #6790, #7872, #215, #3801, #1055, #8486, #3710 ) ) ;
#1302=DIRECTION ( 'NONE',  ( 0.000000000000000000, 0.000000000000000000, 1.000000000000000000 ) ) ;
#1303=AXIS2_PLACEMENT_3D ( 'NONE', #6185, #4630, #9308 ) ;
#1307=EDGE_CURVE ( 'NONE', #3216, #9419, #3578, .T. ) ;
#1309=CARTESIAN_POINT ( 'NONE',  ( 0.000000000000000000, 39.99999999999999289, 0.000000000000000000 ) ) ;
#1310=ORIENTED_EDGE ( 'NONE', *, *, #2619, .F. ) ;
#1313=TOROIDAL_SURFACE ( 'NONE', #220, 33.00000000000000711, 5.000000000000000000 ) ;
#1317=DIRECTION ( 'NONE',  ( -0.000000000000000000, 1.000000000000000000, -0.000000000000000000 ) ) ;
#1319=LINE ( 'NONE', #5173, #4592 ) ;
#1320=ORIENTED_EDGE ( 'NONE', *, *, #2371, .F. ) ;
#1321=CYLINDRICAL_SURFACE ( 'NONE', #4674, 25.00000000000000000 ) ;
#1323=ORIENTED_EDGE ( 'NONE', *, *, #3240, .F. ) ;
#1328=CARTESIAN_POINT ( 'NONE',  ( 0.000000000000000000, 30.99999999999998579, 0.000000000000000000 ) ) ;
#1330=DIRECTION ( 'NONE',  ( 0.000000000000000000, 0.000000000000000000, 1.000000000000000000 ) ) ;
#1332=ORIENTED_EDGE ( 'NONE', *, *, #1217, .T. ) ;
#1334=CARTESIAN_POINT ( 'NONE',  ( 0.000000000000000000, 39.99999999999999289, 0.000000000000000000 ) ) ;
#1335=DIRECTION ( 'NONE',  ( 0.000000000000000000, 1.000000000000000000, 0.000000000000000000 ) ) ;
#1342=CARTESIAN_POINT ( 'NONE',  ( 12.48950176432140680, 54.99999999999999289, 35.88888888888889284 ) ) ;
#1344=CARTESIAN_POINT ( 'NONE',  ( 0.000000000000000000, 39.99999999999999289, 0.000000000000000000 ) ) ;
#1352=CARTESIAN_POINT ( 'NONE',  ( -29.00000000000000355, 0.000000000000000000, -3.999999999999996447 ) ) ;
#1354=DIRECTION ( 'NONE',  ( 0.000000000000000000, -1.000000000000000000, 0.000000000000000000 ) ) ;
#1355=AXIS2_PLACEMENT_3D ( 'NONE', #2964, #6755, #1440 ) ;
#1361=LINE ( 'NONE', #4475, #3620 ) ;
#1362=DIRECTION ( 'NONE',  ( 0.000000000000000000, 0.000000000000000000, 1.000000000000000000 ) ) ;
#1363=ADVANCED_FACE ( 'NONE', ( #6530 ), #8289, .F. ) ;
#1365=AXIS2_PLACEMENT_3D ( 'NONE', #7053, #995, #9202 ) ;
#1367=CIRCLE ( 'NONE', #6878, 2.500000000000002220 ) ;
#1370=PLANE ( 'NONE',  #418 ) ;
#1372=EDGE_CURVE ( 'NONE', #9687, #5003, #1993, .T. ) ;
#1377=DIRECTION ( 'NONE',  ( -0.000000000000000000, -1.000000000000000000, -0.000000000000000000 ) ) ;
#1380=CARTESIAN_POINT ( 'NONE',  ( -33.06426808735054124, 59.99999999999999289, -5.562309845534581854 ) ) ;
#1383=DIRECTION ( 'NONE',  ( 0.000000000000000000, 0.000000000000000000, -1.000000000000000000 ) ) ;
#1384=EDGE_LOOP ( 'NONE', ( #2181, #2570, #7626, #8864 ) ) ;
#1385=B_SPLINE_CURVE_WITH_KNOTS ( 'NONE', 3,
 ( #2336, #1510, #4633, #1560 ),
 .UNSPECIFIED., .F., .F.,
 ( 4, 4 ),
 ( 0.009125339089286721786, 0.009329711147074794264 ),
 .UNSPECIFIED. ) ;
#1389=CARTESIAN_POINT ( 'NONE',  ( -35.43299232931641995, 59.17741350630852537, -4.746722514775166601 ) ) ;
#1390=ORIENTED_EDGE ( 'NONE', *, *, #1902, .F. ) ;
#1391=CARTESIAN_POINT ( 'NONE',  ( 0.000000000000000000, 59.99999999999999289, 0.000000000000000000 ) ) ;
#1394=APPLICATION_CONTEXT ( 'automotive_design' ) ;
#1395=EDGE_LOOP ( 'NONE', ( #7967, #2318, #966, #609 ) ) ;
#1398=LINE ( 'NONE', #7427, #3196 ) ;
#1400=DIRECTION ( 'NONE',  ( 0.000000000000000000, 0.000000000000000000, -1.000000000000000000 ) ) ;
#1402=LINE ( 'NONE', #3020, #5521 ) ;
#1404=ADVANCED_FACE ( 'NONE', ( #3622 ), #8811, .T. ) ;
#1408=DIRECTION ( 'NONE',  ( 0.000000000000000000, 0.000000000000000000, 1.000000000000000000 ) ) ;
#1410=LINE ( 'NONE', #4431, #3241 ) ;
#1415=AXIS2_PLACEMENT_3D ( 'NONE', #2262, #5296, #4611 ) ;
#1416=CIRCLE ( 'NONE', #7249, 38.00000000000000711 ) ;
#1419=ADVANCED_FACE ( 'NONE', ( #5456 ), #4671, .F. ) ;
#1421=EDGE_CURVE ( 'NONE', #1969, #3718, #6693, .T. ) ;
#1426=CARTESIAN_POINT ( 'NONE',  ( -18.58791755254457456, 59.99999999999999289, -23.54759692749571443 ) ) ;
#1429=CIRCLE ( 'NONE', #8212, 30.00000000000000711 ) ;
#1430=CARTESIAN_POINT ( 'NONE',  ( 0.000000000000000000, 39.99999999999999289, 0.000000000000000000 ) ) ;
#1433=ADVANCED_FACE ( 'NONE', ( #6917 ), #3769, .F. ) ;
#1437=VERTEX_POINT ( 'NONE', #5979 ) ;
#1438=CARTESIAN_POINT ( 'NONE',  ( 35.03233509200964590, 59.17868483491578502, 7.112484670352360538 ) ) ;
#1439=ORIENTED_EDGE ( 'NONE', *, *, #6960, .F. ) ;
#1440=DIRECTION ( 'NONE',  ( 0.000000000000000000, -0.000000000000000000, 1.000000000000000000 ) ) ;
#1441=ORIENTED_EDGE ( 'NONE', *, *, #4415, .F. ) ;
#1445=CARTESIAN_POINT ( 'NONE',  ( 0.000000000000000000, 1.000000000000014655, 0.000000000000000000 ) ) ;
#1449=ORIENTED_EDGE ( 'NONE', *, *, #8908, .F. ) ;
#1453=DIRECTION ( 'NONE',  ( 0.000000000000000000, -0.000000000000000000, 1.000000000000000000 ) ) ;
#1454=AXIS2_PLACEMENT_3D ( 'NONE', #5080, #4445, #31 ) ;
#1461=EDGE_CURVE ( 'NONE', #4111, #7715, #7706, .T. ) ;
#1462=DIRECTION ( 'NONE',  ( 0.000000000000000000, 0.000000000000000000, 1.000000000000000000 ) ) ;
#1467=VERTEX_POINT ( 'NONE', #78 ) ;
#1468=LINE ( 'NONE', #8296, #5094 ) ;
#1470=EDGE_LOOP ( 'NONE', ( #2860, #4315, #52, #1310 ) ) ;
#1471=EDGE_CURVE ( 'NONE', #9386, #7724, #9718, .T. ) ;
#1478=VERTEX_POINT ( 'NONE', #2327 ) ;
#1480=VECTOR ( 'NONE', #2008, 1000.000000000000000 ) ;
#1481=FACE_OUTER_BOUND ( 'NONE', #5832, .T. ) ;
#1485=FACE_OUTER_BOUND ( 'NONE', #3829, .T. ) ;
#1488=DIRECTION ( 'NONE',  ( 0.000000000000000000, 0.000000000000000000, 1.000000000000000000 ) ) ;
#1490=CARTESIAN_POINT ( 'NONE',  ( -12.43339847825378719, 59.99999999999999289, 35.90836395996003461 ) ) ;
#1491=DIRECTION ( 'NONE',  ( 0.9449569463147373671, -0.000000000000000000, 0.3271946967961530395 ) ) ;
#1492=AXIS2_PLACEMENT_3D ( 'NONE', #5946, #9563, #3628 ) ;
#1493=EDGE_LOOP ( 'NONE', ( #5313, #1972, #8810, #7065, #865, #8191, #3523, #2144 ) ) ;
#1494=CARTESIAN_POINT ( 'NONE',  ( -6.957283601945606577, 59.12244502749634023, 35.14908888799237729 ) ) ;
#1501=( NAMED_UNIT ( * ) SI_UNIT ( $, .STERADIAN. ) SOLID_ANGLE_UNIT ( ) );
#1502=DIRECTION ( 'NONE',  ( -0.7071067811865573427, 0.7071067811865376918, 1.533293416683393860E-16 ) ) ;
#1503=B_SPLINE_CURVE_WITH_KNOTS ( 'NONE', 3,
 ( #7866, #2556, #1142, #2609, #407, #1920 ),
 .UNSPECIFIED., .F., .F.,
 ( 4, 2, 4 ),
 ( 0.000000000000000000, 0.0005212762617847652939, 0.001042552523569530588 ),
 .UNSPECIFIED. ) ;
#1504=CARTESIAN_POINT ( 'NONE',  ( 2.204364238465235033E-15, 1.000000000000014655, 17.99999999999999645 ) ) ;
#1510=CARTESIAN_POINT ( 'NONE',  ( -32.99503133754566875, 59.99860354191589806, -3.062309845534580077 ) ) ;
#1511=ORIENTED_EDGE ( 'NONE', *, *, #1307, .T. ) ;
#1513=LINE ( 'NONE', #827, #8456 ) ;
#1514=DIRECTION ( 'NONE',  ( 0.000000000000000000, 0.000000000000000000, 1.000000000000000000 ) ) ;
#1521=VECTOR ( 'NONE', #4246, 1000.000000000000000 ) ;
#1524=ORIENTED_EDGE ( 'NONE', *, *, #7025, .F. ) ;
#1527=VERTEX_POINT ( 'NONE', #365 ) ;
#1533=EDGE_CURVE ( 'NONE', #2965, #1437, #1818, .T. ) ;
#1541=ORIENTED_EDGE ( 'NONE', *, *, #8719, .F. ) ;
#1543=ORIENTED_EDGE ( 'NONE', *, *, #9095, .T. ) ;
#1544=EDGE_CURVE ( 'NONE', #4065, #6089, #8561, .T. ) ;
#1548=EDGE_CURVE ( 'NONE', #7738, #167, #6424, .T. ) ;
#1550=EDGE_CURVE ( 'NONE', #1104, #4952, #1930, .T. ) ;
#1553=EDGE_CURVE ( 'NONE', #1933, #9639, #1975, .T. ) ;
#1558=LINE ( 'NONE', #5466, #5093 ) ;
#1560=CARTESIAN_POINT ( 'NONE',  ( -32.85680095556730862, 59.99999999999999289, -3.070933240276025877 ) ) ;
#1561=DIRECTION ( 'NONE',  ( 0.000000000000000000, 0.000000000000000000, -1.000000000000000000 ) ) ;
#1564=CARTESIAN_POINT ( 'NONE',  ( 0.000000000000000000, 30.00000000000000000, 0.000000000000000000 ) ) ;
#1566=CARTESIAN_POINT ( 'NONE',  ( 33.00000000000000711, 54.99999999999999289, 1.152188841818234638E-13 ) ) ;
#1570=DIRECTION ( 'NONE',  ( 0.000000000000000000, 0.000000000000000000, 1.000000000000000000 ) ) ;
#1571=ORIENTED_EDGE ( 'NONE', *, *, #7347, .F. ) ;
#1572=CARTESIAN_POINT ( 'NONE',  ( 4.000000000000008882, 30.00000000000000000, 29.00000000000000355 ) ) ;
#1573=AXIS2_PLACEMENT_3D ( 'NONE', #3959, #5445, #2315 ) ;
#1574=CIRCLE ( 'NONE', #9304, 38.00000000000000000 ) ;
#1578=EDGE_LOOP ( 'NONE', ( #4422, #3915, #177, #9494, #3197 ) ) ;
#1582=PLANE ( 'NONE',  #1927 ) ;
#1584=DIRECTION ( 'NONE',  ( 0.000000000000000000, 0.000000000000000000, 1.000000000000000000 ) ) ;
#1585=ORIENTED_EDGE ( 'NONE', *, *, #6897, .T. ) ;
#1588=ADVANCED_FACE ( 'NONE', ( #7060 ), #8708, .T. ) ;
#1589=ORIENTED_EDGE ( 'NONE', *, *, #1841, .F. ) ;
#1591=CARTESIAN_POINT ( 'NONE',  ( -24.67792535850613334, 28.99999999999997158, 4.000000000000009770 ) ) ;
#1592=PLANE ( 'NONE',  #6541 ) ;
#1593=DIRECTION ( 'NONE',  ( 0.3286710990611141914, 0.000000000000000000, 0.9444444444444359821 ) ) ;
#1594=CIRCLE ( 'NONE', #2048, 38.00000000000000711 ) ;
#1597=CARTESIAN_POINT ( 'NONE',  ( 29.00000000000000355, 28.99999999999997158, -4.000000000000007105 ) ) ;
#1600=ORIENTED_EDGE ( 'NONE', *, *, #3220, .F. ) ;
#1603=ORIENTED_EDGE ( 'NONE', *, *, #4430, .T. ) ;
#1606=EDGE_CURVE ( 'NONE', #2818, #7534, #9471, .T. ) ;
#1611=ORIENTED_EDGE ( 'NONE', *, *, #831, .F. ) ;
#1612=CARTESIAN_POINT ( 'NONE',  ( 0.000000000000000000, 59.99999999999999289, 38.00000000000000711 ) ) ;
#1616=CARTESIAN_POINT ( 'NONE',  ( -5.562309845534584518, 49.99999999999999289, 30.56426808735054124 ) ) ;
#1618=PLANE ( 'NONE',  #8218 ) ;
#1619=DIRECTION ( 'NONE',  ( 0.000000000000000000, 1.000000000000000000, 0.000000000000000000 ) ) ;
#1622=VECTOR ( 'NONE', #3734, 1000.000000000000000 ) ;
#1624=ORIENTED_EDGE ( 'NONE', *, *, #1897, .T. ) ;
#1625=DIRECTION ( 'NONE',  ( 0.000000000000000000, 0.000000000000000000, -1.000000000000000000 ) ) ;
#1627=AXIS2_PLACEMENT_3D ( 'NONE', #2168, #1491, #8069 ) ;
#1631=DIRECTION ( 'NONE',  ( 0.000000000000000000, 0.000000000000000000, 1.000000000000000000 ) ) ;
#1634=ORIENTED_EDGE ( 'NONE', *, *, #7005, .F. ) ;
#1636=CARTESIAN_POINT ( 'NONE',  ( 24.96033808169876878, 29.33187429063046991, 4.331874290630486790 ) ) ;
#1648=AXIS2_PLACEMENT_3D ( 'NONE', #6876, #1502, #3121 ) ;
#1652=VERTEX_POINT ( 'NONE', #1342 ) ;
#1653=DIRECTION ( 'NONE',  ( -0.000000000000000000, -1.000000000000000000, -0.000000000000000000 ) ) ;
#1658=ORIENTED_EDGE ( 'NONE', *, *, #9330, .T. ) ;
#1660=ADVANCED_FACE ( 'NONE', ( #8753 ), #2118, .F. ) ;
#1663=ADVANCED_FACE ( 'NONE', ( #4367 ), #3465, .F. ) ;
#1668=VECTOR ( 'NONE', #4122, 1000.000000000000114 ) ;
#1673=VECTOR ( 'NONE', #4886, 1000.000000000000000 ) ;
#1674=AXIS2_PLACEMENT_3D ( 'NONE', #4891, #6361, #2501 ) ;
#1676=EDGE_CURVE ( 'NONE', #5781, #7004, #8605, .T. ) ;
#1677=EDGE_LOOP ( 'NONE', ( #2866, #1524, #8500, #3556 ) ) ;
#1682=CIRCLE ( 'NONE', #1213, 33.00000000000000711 ) ;
#1687=CARTESIAN_POINT ( 'NONE',  ( -31.18357922838634266, 54.99999999999999289, -10.79742499427304558 ) ) ;
#1692=VERTEX_POINT ( 'NONE', #4310 ) ;
#1694=EDGE_CURVE ( 'NONE', #5598, #9259, #9709, .T. ) ;
#1696=ORIENTED_EDGE ( 'NONE', *, *, #2990, .F. ) ;
#1697=DIRECTION ( 'NONE',  ( -0.9449569463147371451, 0.000000000000000000, -0.3271946967961539277 ) ) ;
#1700=DIRECTION ( 'NONE',  ( 0.000000000000000000, 0.000000000000000000, 1.000000000000000000 ) ) ;
#1701=CARTESIAN_POINT ( 'NONE',  ( -28.34870838944214455, 59.99999999999999289, -9.815840903884556212 ) ) ;
#1704=DIRECTION ( 'NONE',  ( 0.000000000000000000, 1.000000000000000000, 0.000000000000000000 ) ) ;
#1707=EDGE_CURVE ( 'NONE', #1097, #5855, #5606, .T. ) ;
#1709=CARTESIAN_POINT ( 'NONE',  ( 7.548108395552117322, 59.38382381638697893, -34.59619211116746840 ) ) ;
#1721=ORIENTED_EDGE ( 'NONE', *, *, #7076, .F. ) ;
#1722=EDGE_CURVE ( 'NONE', #9059, #1935, #5195, .T. ) ;
#1730=DIRECTION ( 'NONE',  ( 0.000000000000000000, 1.000000000000000000, 0.000000000000000000 ) ) ;
#1735=DIRECTION ( 'NONE',  ( 0.000000000000000000, 1.000000000000000000, 0.000000000000000000 ) ) ;
#1741=ORIENTED_EDGE ( 'NONE', *, *, #1606, .F. ) ;
#1742=CARTESIAN_POINT ( 'NONE',  ( -34.69710844949434403, 59.33700357310857498, -7.462191142828213053 ) ) ;
#1743=ORIENTED_EDGE ( 'NONE', *, *, #3291, .T. ) ;
#1744=CARTESIAN_POINT ( 'NONE',  ( 33.72085295419949347, 59.72647237447257851, 7.995677060003923309 ) ) ;
#1748=DIRECTION ( 'NONE',  ( 0.000000000000000000, 1.000000000000000000, 0.000000000000000000 ) ) ;
#1752=VERTEX_POINT ( 'NONE', #3916 ) ;
#1754=DIRECTION ( 'NONE',  ( 3.491481338843134539E-15, -0.000000000000000000, -1.000000000000000000 ) ) ;
#1757=DIRECTION ( 'NONE',  ( -0.9444444444444360931, -0.000000000000000000, 0.3286710990611142469 ) ) ;
#1759=LINE ( 'NONE', #151, #7245 ) ;
#1761=CARTESIAN_POINT ( 'NONE',  ( -35.90836395996003461, 39.99999999999999289, -12.43339847825377475 ) ) ;
#1762=ORIENTED_EDGE ( 'NONE', *, *, #6843, .F. ) ;
#1763=DIRECTION ( 'NONE',  ( -0.000000000000000000, 1.000000000000000000, -0.000000000000000000 ) ) ;
#1765=ORIENTED_EDGE ( 'NONE', *, *, #280, .F. ) ;
#1768=CARTESIAN_POINT ( 'NONE',  ( 0.000000000000000000, 0.000000000000000000, -29.00000000000000355 ) ) ;
#1776=VERTEX_POINT ( 'NONE', #5967 ) ;
#1779=CYLINDRICAL_SURFACE ( 'NONE', #9255, 30.00000000000001066 ) ;
#1787=CARTESIAN_POINT ( 'NONE',  ( -35.29563341415538247, 59.05475394944627965, -6.702038549863909012 ) ) ;
#1789=VERTEX_POINT ( 'NONE', #4657 ) ;
#1790=DIRECTION ( 'NONE',  ( -0.000000000000000000, -1.000000000000000000, -0.000000000000000000 ) ) ;
#1795=CYLINDRICAL_SURFACE ( 'NONE', #844, 38.00000000000000711 ) ;
#1796=CIRCLE ( 'NONE', #9227, 30.00000000000000711 ) ;
#1801=CARTESIAN_POINT ( 'NONE',  ( -20.00000000000019185, 19.99999999999990763, 4.999999999999814371 ) ) ;
#1804=AXIS2_PLACEMENT_3D ( 'NONE', #4884, #3448, #9525 ) ;
#1805=AXIS2_PLACEMENT_3D ( 'NONE', #1328, #9480, #1283 ) ;
#1806=CYLINDRICAL_SURFACE ( 'NONE', #6458, 38.00000000000000711 ) ;
#1807=CARTESIAN_POINT ( 'NONE',  ( 30.00000000000000711, 30.00000000000000000, 0.000000000000000000 ) ) ;
#1814=CIRCLE ( 'NONE', #5605, 2.500000000000002220 ) ;
#1816=FACE_OUTER_BOUND ( 'NONE', #7478, .T. ) ;
#1817=DIRECTION ( 'NONE',  ( 6.982962677686269866E-15, -0.000000000000000000, -1.000000000000000000 ) ) ;
#1818=CIRCLE ( 'NONE', #6856, 30.00000000000001066 ) ;
#1822=AXIS2_PLACEMENT_3D ( 'NONE', #1010, #6430, #7830 ) ;
#1823=DIRECTION ( 'NONE',  ( 2.168404344971006649E-16, -0.000000000000000000, 1.000000000000000000 ) ) ;
#1824=DIRECTION ( 'NONE',  ( -0.000000000000000000, -1.000000000000000000, -0.000000000000000000 ) ) ;
#1830=CARTESIAN_POINT ( 'NONE',  ( -33.06426808735054124, 49.99999999999999289, -5.562309845534581854 ) ) ;
#1835=LINE ( 'NONE', #413, #6334 ) ;
#1841=EDGE_CURVE ( 'NONE', #6883, #9419, #8253, .T. ) ;
#1842=VERTEX_POINT ( 'NONE', #3711 ) ;
#1847=DIRECTION ( 'NONE',  ( 0.000000000000000000, 0.000000000000000000, -1.000000000000000000 ) ) ;
#1855=DIRECTION ( 'NONE',  ( 0.000000000000000000, 1.000000000000000000, 0.000000000000000000 ) ) ;
#1857=DIRECTION ( 'NONE',  ( 0.000000000000000000, 0.000000000000000000, 1.000000000000000000 ) ) ;
#1863=PRODUCT_DEFINITION ( 'UNKNOWN', '', #2057, #6030 ) ;
#1864=VERTEX_POINT ( 'NONE', #4507 ) ;
#1867=CARTESIAN_POINT ( 'NONE',  ( 28.33333333333337833, 59.99999999999999289, -9.860132971832594961 ) ) ;
#1869=CARTESIAN_POINT ( 'NONE',  ( -30.00000000000001066, 59.99999999999999289, -3.252551416882082410E-13 ) ) ;
#1875=AXIS2_PLACEMENT_3D ( 'NONE', #8965, #621, #2879 ) ;
#1876=DIRECTION ( 'NONE',  ( -0.000000000000000000, -1.000000000000000000, -0.000000000000000000 ) ) ;
#1877=EDGE_CURVE ( 'NONE', #6765, #7824, #1110, .T. ) ;
#1881=DIRECTION ( 'NONE',  ( 0.000000000000000000, 0.000000000000000000, 1.000000000000000000 ) ) ;
#1886=AXIS2_PLACEMENT_3D ( 'NONE', #5167, #8171, #9065 ) ;
#1890=CARTESIAN_POINT ( 'NONE',  ( 0.000000000000000000, 59.99999999999999289, 0.000000000000000000 ) ) ;
#1893=ORIENTED_EDGE ( 'NONE', *, *, #1548, .F. ) ;
#1896=PLANE ( 'NONE',  #2258 ) ;
#1897=EDGE_CURVE ( 'NONE', #6355, #7824, #7467, .T. ) ;
#1900=DIRECTION ( 'NONE',  ( -0.000000000000000000, -1.000000000000000000, -0.000000000000000000 ) ) ;
#1902=EDGE_CURVE ( 'NONE', #6149, #8330, #3407, .T. ) ;
#1906=CARTESIAN_POINT ( 'NONE',  ( 0.000000000000000000, 39.99999999999999289, -30.00000000000000711 ) ) ;
#1907=ORIENTED_EDGE ( 'NONE', *, *, #8723, .F. ) ;
#1908=DIRECTION ( 'NONE',  ( 1.000000000000000000, 0.000000000000000000, 3.491481338843134539E-15 ) ) ;
#1909=CARTESIAN_POINT ( 'NONE',  ( 0.000000000000000000, 30.99999999999998579, 40.00000000000000711 ) ) ;
#1915=DIRECTION ( 'NONE',  ( 0.000000000000000000, 0.000000000000000000, 1.000000000000000000 ) ) ;
#1917=ORIENTED_EDGE ( 'NONE', *, *, #810, .F. ) ;
#1918=LINE ( 'NONE', #1187, #7645 ) ;
#1920=CARTESIAN_POINT ( 'NONE',  ( 33.06426808735053413, 59.89212256466219486, 8.062309845534588959 ) ) ;
#1922=AXIS2_PLACEMENT_3D ( 'NONE', #2760, #5786, #6801 ) ;
#1924=DIRECTION ( 'NONE',  ( 0.000000000000000000, 0.000000000000000000, 1.000000000000000000 ) ) ;
#1925=CARTESIAN_POINT ( 'NONE',  ( 0.000000000000000000, 37.99999999999996447, 0.000000000000000000 ) ) ;
#1926=ADVANCED_FACE ( 'NONE', ( #9247 ), #3253, .F. ) ;
#1927=AXIS2_PLACEMENT_3D ( 'NONE', #7561, #2406, #899 ) ;
#1930=LINE ( 'NONE', #6226, #9242 ) ;
#1933=VERTEX_POINT ( 'NONE', #403 ) ;
#1935=VERTEX_POINT ( 'NONE', #5443 ) ;
#1937=CIRCLE ( 'NONE', #9206, 37.99999999999999289 ) ;
#1941=EDGE_LOOP ( 'NONE', ( #4355, #7203, #6076, #9375 ) ) ;
#1943=EDGE_LOOP ( 'NONE', ( #2612, #3823, #430, #7018, #406 ) ) ;
#1944=FACE_BOUND ( 'NONE', #6139, .T. ) ;
#1948=DIRECTION ( 'NONE',  ( 0.000000000000000000, 1.000000000000000000, 0.000000000000000000 ) ) ;
#1951=EDGE_CURVE ( 'NONE', #3761, #8698, #3078, .T. ) ;
#1956=DIRECTION ( 'NONE',  ( 0.7849198975831892522, 0.000000000000000000, -0.6195972517514870548 ) ) ;
#1958=ORIENTED_EDGE ( 'NONE', *, *, #9216, .T. ) ;
#1959=PLANE ( 'NONE',  #3651 ) ;
#1960=CARTESIAN_POINT ( 'NONE',  ( -4.000000000000005329, 0.000000000000000000, -24.67792535850613334 ) ) ;
#1962=PLANE ( 'NONE',  #1454 ) ;
#1963=AXIS2_PLACEMENT_3D ( 'NONE', #3744, #3794, #1462 ) ;
#1964=EDGE_CURVE ( 'NONE', #7838, #4449, #4159, .T. ) ;
#1969=VERTEX_POINT ( 'NONE', #5536 ) ;
#1972=ORIENTED_EDGE ( 'NONE', *, *, #7129, .F. ) ;
#1974=AXIS2_PLACEMENT_3D ( 'NONE', #5146, #1335, #9536 ) ;
#1975=CIRCLE ( 'NONE', #5304, 26.00000000000000355 ) ;
#1976=DIRECTION ( 'NONE',  ( 0.000000000000000000, 0.000000000000000000, 1.000000000000000000 ) ) ;
#1977=CIRCLE ( 'NONE', #8134, 26.00000000000000355 ) ;
#1980=VERTEX_POINT ( 'NONE', #1869 ) ;
#1981=CARTESIAN_POINT ( 'NONE',  ( -33.89029069002005912, 59.89318186371823316, -3.196943324609351045 ) ) ;
#1984=CARTESIAN_POINT ( 'NONE',  ( 35.47893788052810038, 58.98370868798952671, 6.231324730575376059 ) ) ;
#1989=LINE ( 'NONE', #323, #8924 ) ;
#1990=DIRECTION ( 'NONE',  ( -0.000000000000000000, -1.000000000000000000, -0.000000000000000000 ) ) ;
#1992=VERTEX_POINT ( 'NONE', #7712 ) ;
#1993=LINE ( 'NONE', #2083, #4983 ) ;
#1997=DIRECTION ( 'NONE',  ( 0.000000000000000000, -0.000000000000000000, 1.000000000000000000 ) ) ;
#2002=CARTESIAN_POINT ( 'NONE',  ( -33.06426808735053413, 59.89212256466219486, -8.062309845534585406 ) ) ;
#2004=ORIENTED_EDGE ( 'NONE', *, *, #8668, .F. ) ;
#2005=DIRECTION ( 'NONE',  ( 7.666467083416968066E-17, -0.7071067811865378028, 0.7071067811865572317 ) ) ;
#2006=CARTESIAN_POINT ( 'NONE',  ( 35.90836395996004171, 59.99999999999999289, 12.43339847825378186 ) ) ;
#2007=ADVANCED_FACE ( 'NONE', ( #7804 ), #3303, .T. ) ;
#2008=DIRECTION ( 'NONE',  ( -0.000000000000000000, -1.000000000000000000, -0.000000000000000000 ) ) ;
#2009=LINE ( 'NONE', #2979, #2871 ) ;
#2012=CARTESIAN_POINT ( 'NONE',  ( 4.000000000000002665, 0.000000000000000000, -8.673617379884032514E-16 ) ) ;
#2018=DIRECTION ( 'NONE',  ( 0.000000000000000000, 1.000000000000000000, 0.000000000000000000 ) ) ;
#2019=DIRECTION ( 'NONE',  ( 0.000000000000000000, 0.000000000000000000, 1.000000000000000000 ) ) ;
#2022=ORIENTED_EDGE ( 'NONE', *, *, #280, .T. ) ;
#2028=ORIENTED_EDGE ( 'NONE', *, *, #5393, .T. ) ;
#2030=DIRECTION ( 'NONE',  ( -0.000000000000000000, -1.000000000000000000, -0.000000000000000000 ) ) ;
#2031=LINE ( 'NONE', #3670, #7621 ) ;
#2034=ORIENTED_EDGE ( 'NONE', *, *, #8682, .F. ) ;
#2037=EDGE_LOOP ( 'NONE', ( #8017, #5431, #7356, #1261 ) ) ;
#2038=CYLINDRICAL_SURFACE ( 'NONE', #2725, 30.00000000000000711 ) ;
#2041=FACE_OUTER_BOUND ( 'NONE', #2679, .T. ) ;
#2043=AXIS2_PLACEMENT_3D ( 'NONE', #4080, #6337, #9358 ) ;
#2044=DIRECTION ( 'NONE',  ( 0.000000000000000000, 0.000000000000000000, -1.000000000000000000 ) ) ;
#2048=AXIS2_PLACEMENT_3D ( 'NONE', #8635, #4923, #1857 ) ;
#2052=DIRECTION ( 'NONE',  ( 0.3286710990611141914, 0.000000000000000000, 0.9444444444444359821 ) ) ;
#2053=CARTESIAN_POINT ( 'NONE',  ( 30.00000000000000711, 39.99999999999999289, 1.047444401652940259E-13 ) ) ;
#2056=CARTESIAN_POINT ( 'NONE',  ( 9.815840903884561541, 59.99999999999999289, -28.34870838944214100 ) ) ;
#2057=PRODUCT_DEFINITION_FORMATION_WITH_SPECIFIED_SOURCE ( 'ANY', '', #6053, .NOT_KNOWN. ) ;
#2058=ORIENTED_EDGE ( 'NONE', *, *, #1461, .F. ) ;
#2061=ORIENTED_EDGE ( 'NONE', *, *, #5948, .F. ) ;
#2062=CARTESIAN_POINT ( 'NONE',  ( 0.000000000000000000, 59.99999999999999289, 0.000000000000000000 ) ) ;
#2075=CARTESIAN_POINT ( 'NONE',  ( -5.562309845534584518, 49.99999999999999289, 33.06426808735054124 ) ) ;
#2076=ORIENTED_EDGE ( 'NONE', *, *, #8696, .F. ) ;
#2079=AXIS2_PLACEMENT_3D ( 'NONE', #6062, #3853, #6160 ) ;
#2080=DIRECTION ( 'NONE',  ( 0.000000000000000000, 0.000000000000000000, 1.000000000000000000 ) ) ;
#2082=ORIENTED_EDGE ( 'NONE', *, *, #290, .T. ) ;
#2083=CARTESIAN_POINT ( 'NONE',  ( 29.82695610816121956, 59.99999999999999289, -23.54469556655648077 ) ) ;
#2084=EDGE_CURVE ( 'NONE', #9419, #6457, #5819, .T. ) ;
#2087=AXIS2_PLACEMENT_3D ( 'NONE', #8037, #1277, #450 ) ;
#2090=CARTESIAN_POINT ( 'NONE',  ( -23.54469556655647722, 59.99999999999999289, -29.82695610816121956 ) ) ;
#2092=ORIENTED_EDGE ( 'NONE', *, *, #5656, .T. ) ;
#2093=DIRECTION ( 'NONE',  ( 0.000000000000000000, 0.000000000000000000, 1.000000000000000000 ) ) ;
#2094=CARTESIAN_POINT ( 'NONE',  ( 28.34870838944214100, 39.99999999999999289, 9.815840903884559765 ) ) ;
#2099=ADVANCED_FACE ( 'NONE', ( #5862 ), #8591, .T. ) ;
#2100=CIRCLE ( 'NONE', #2743, 17.99999999999999645 ) ;
#2101=DIRECTION ( 'NONE',  ( -0.9449569463147374782, 0.000000000000000000, -0.3271946967961530950 ) ) ;
#2102=ORIENTED_EDGE ( 'NONE', *, *, #690, .T. ) ;
#2106=CIRCLE ( 'NONE', #870, 33.00000000000000711 ) ;
#2108=CARTESIAN_POINT ( 'NONE',  ( 4.000000000000001776, 28.99999999999997158, -24.67792535850613334 ) ) ;
#2111=EDGE_LOOP ( 'NONE', ( #5621, #2642, #1441, #9501, #1133, #2058, #8657 ) ) ;
#2118=CYLINDRICAL_SURFACE ( 'NONE', #7340, 30.00000000000000711 ) ;
#2120=CARTESIAN_POINT ( 'NONE',  ( 9.860132971832495485, 59.99999999999999289, 28.33333333333341031 ) ) ;
#2121=ORIENTED_EDGE ( 'NONE', *, *, #6525, .F. ) ;
#2124=AXIS2_PLACEMENT_3D ( 'NONE', #8654, #2709, #8559 ) ;
#2127=AXIS2_PLACEMENT_3D ( 'NONE', #317, #5507, #8514 ) ;
#2129=TOROIDAL_SURFACE ( 'NONE', #105, 33.00000000000000711, 5.000000000000000000 ) ;
#2131=CARTESIAN_POINT ( 'NONE',  ( 0.000000000000000000, 37.99999999999996447, 0.000000000000000000 ) ) ;
#2133=VECTOR ( 'NONE', #6212, 1000.000000000000000 ) ;
#2134=ORIENTED_EDGE ( 'NONE', *, *, #7025, .T. ) ;
#2139=EDGE_CURVE ( 'NONE', #4095, #8510, #6049, .T. ) ;
#2142=ADVANCED_FACE ( 'NONE', ( #9527 ), #5780, .F. ) ;
#2144=ORIENTED_EDGE ( 'NONE', *, *, #9146, .F. ) ;
#2146=CARTESIAN_POINT ( 'NONE',  ( -32.05305536707737701, 59.99999999999999289, -7.848671329280701769 ) ) ;
#2147=FACE_OUTER_BOUND ( 'NONE', #8893, .T. ) ;
#2151=DIRECTION ( 'NONE',  ( 0.000000000000000000, -0.000000000000000000, 1.000000000000000000 ) ) ;
#2152=VERTEX_POINT ( 'NONE', #7953 ) ;
#2155=ORIENTED_EDGE ( 'NONE', *, *, #6224, .F. ) ;
#2160=DIRECTION ( 'NONE',  ( 1.000000000000000000, 0.000000000000000000, -0.000000000000000000 ) ) ;
#2161=ORIENTED_EDGE ( 'NONE', *, *, #2427, .T. ) ;
#2162=DIRECTION ( 'NONE',  ( 0.000000000000000000, 1.000000000000000000, 0.000000000000000000 ) ) ;
#2164=PLANE ( 'NONE',  #1355 ) ;
#2168=CARTESIAN_POINT ( 'NONE',  ( 10.79742499427305269, 54.99999999999999289, -31.18357922838633911 ) ) ;
#2171=ADVANCED_FACE ( 'NONE', ( #5679 ), #5136, .T. ) ;
#2176=( LENGTH_UNIT ( ) NAMED_UNIT ( * ) SI_UNIT ( .MILLI., .METRE. ) );
#2180=EDGE_CURVE ( 'NONE', #1980, #5194, #8044, .T. ) ;
#2181=ORIENTED_EDGE ( 'NONE', *, *, #7636, .F. ) ;
#2184=EDGE_CURVE ( 'NONE', #6883, #6218, #1918, .T. ) ;
#2187=AXIS2_PLACEMENT_3D ( 'NONE', #9333, #8222, #401 ) ;
#2191=EDGE_CURVE ( 'NONE', #2351, #5863, #6842, .T. ) ;
#2195=ORIENTED_EDGE ( 'NONE', *, *, #223, .F. ) ;
#2197=AXIS2_PLACEMENT_3D ( 'NONE', #9707, #7436, #2934 ) ;
#2204=VERTEX_POINT ( 'NONE', #2 ) ;
#2207=LINE ( 'NONE', #9739, #4190 ) ;
#2208=VERTEX_POINT ( 'NONE', #6741 ) ;
#2209=PLANE ( 'NONE',  #5620 ) ;
#2213=DIRECTION ( 'NONE',  ( 0.000000000000000000, -1.000000000000000000, 0.000000000000000000 ) ) ;
#2214=AXIS2_PLACEMENT_3D ( 'NONE', #1430, #8841, #8010 ) ;
#2216=ORIENTED_EDGE ( 'NONE', *, *, #3039, .T. ) ;
#2217=CARTESIAN_POINT ( 'NONE',  ( -5.987883466156522339, 58.97190912209828895, 35.53684633323566544 ) ) ;
#2219=ORIENTED_EDGE ( 'NONE', *, *, #8815, .T. ) ;
#2225=CONICAL_SURFACE ( 'NONE', #7765, 26.00000000000000355, 0.7853981633974346233 ) ;
#2227=VECTOR ( 'NONE', #5231, 1000.000000000000000 ) ;
#2241=AXIS2_PLACEMENT_3D ( 'NONE', #687, #1282, #4297 ) ;
#2244=VERTEX_POINT ( 'NONE', #6052 ) ;
#2247=ORIENTED_EDGE ( 'NONE', *, *, #2427, .F. ) ;
#2252=CIRCLE ( 'NONE', #8902, 26.00000000000000355 ) ;
#2254=ORIENTED_EDGE ( 'NONE', *, *, #3166, .T. ) ;
#2255=EDGE_CURVE ( 'NONE', #167, #2517, #1796, .T. ) ;
#2258=AXIS2_PLACEMENT_3D ( 'NONE', #1165, #3524, #8721 ) ;
#2262=CARTESIAN_POINT ( 'NONE',  ( 0.000000000000000000, 59.99999999999999289, 0.000000000000000000 ) ) ;
#2270=DIRECTION ( 'NONE',  ( 0.000000000000000000, 1.000000000000000000, -0.000000000000000000 ) ) ;
#2271=VECTOR ( 'NONE', #4850, 1000.000000000000000 ) ;
#2279=ORIENTED_EDGE ( 'NONE', *, *, #3349, .T. ) ;
#2282=LINE ( 'NONE', #5316, #2435 ) ;
#2284=CIRCLE ( 'NONE', #1974, 17.99999999999999645 ) ;
#2288=CARTESIAN_POINT ( 'NONE',  ( -10.84614626901596601, 59.99999999999999289, -31.16666666666667851 ) ) ;
#2289=CARTESIAN_POINT ( 'NONE',  ( -4.861949598180842713, 59.13521925290943670, 35.48792514263537612 ) ) ;
#2290=ORIENTED_EDGE ( 'NONE', *, *, #4810, .F. ) ;
#2291=DIRECTION ( 'NONE',  ( -0.000000000000000000, -1.000000000000000000, -0.000000000000000000 ) ) ;
#2299=DIRECTION ( 'NONE',  ( 0.000000000000000000, 1.000000000000000000, 0.000000000000000000 ) ) ;
#2300=ADVANCED_FACE ( 'NONE', ( #840 ), #6694, .T. ) ;
#2301=AXIS2_PLACEMENT_3D ( 'NONE', #3294, #4841, #6257 ) ;
#2304=ORIENTED_EDGE ( 'NONE', *, *, #5533, .F. ) ;
#2305=LINE ( 'NONE', #8984, #374 ) ;
#2307=ORIENTED_EDGE ( 'NONE', *, *, #5529, .F. ) ;
#2315=DIRECTION ( 'NONE',  ( 0.3286710990610906546, 0.000000000000000000, 0.9444444444444440867 ) ) ;
#2317=EDGE_CURVE ( 'NONE', #7738, #1992, #5896, .T. ) ;
#2318=ORIENTED_EDGE ( 'NONE', *, *, #7337, .T. ) ;
#2320=EDGE_CURVE ( 'NONE', #9368, #6765, #2252, .T. ) ;
#2324=DIRECTION ( 'NONE',  ( 0.000000000000000000, -0.000000000000000000, 1.000000000000000000 ) ) ;
#2326=ORIENTED_EDGE ( 'NONE', *, *, #4204, .F. ) ;
#2327=CARTESIAN_POINT ( 'NONE',  ( 9.860132971832495485, 39.99999999999999289, 28.33333333333341031 ) ) ;
#2328=CARTESIAN_POINT ( 'NONE',  ( -4.000000000000001776, 0.000000000000000000, 4.336808689942015271E-16 ) ) ;
#2336=CARTESIAN_POINT ( 'NONE',  ( -33.06426808735054124, 59.99576382555915899, -3.062309845534580077 ) ) ;
#2338=VERTEX_POINT ( 'NONE', #152 ) ;
#2340=CARTESIAN_POINT ( 'NONE',  ( 3.619905045646671926, 59.65318172148984388, -34.64718077370495308 ) ) ;
#2347=AXIS2_PLACEMENT_3D ( 'NONE', #8029, #1265, #6535 ) ;
#2348=DIRECTION ( 'NONE',  ( 0.000000000000000000, 1.000000000000000000, 0.000000000000000000 ) ) ;
#2351=VERTEX_POINT ( 'NONE', #9371 ) ;
#2352=CARTESIAN_POINT ( 'NONE',  ( 29.00000000000000355, 28.99999999999997158, -4.000000000000007105 ) ) ;
#2357=CARTESIAN_POINT ( 'NONE',  ( -33.06426808735054124, 49.99999999999999289, -5.562309845534581854 ) ) ;
#2364=ORIENTED_EDGE ( 'NONE', *, *, #9216, .F. ) ;
#2368=DIRECTION ( 'NONE',  ( 0.000000000000000000, 0.000000000000000000, 1.000000000000000000 ) ) ;
#2369=CARTESIAN_POINT ( 'NONE',  ( 24.67792535850613334, 28.99999999999997158, -4.000000000000006217 ) ) ;
#2371=EDGE_CURVE ( 'NONE', #22, #8061, #9690, .T. ) ;
#2372=EDGE_CURVE ( 'NONE', #1467, #3887, #5524, .T. ) ;
#2375=CARTESIAN_POINT ( 'NONE',  ( 32.92587516511807166, 59.99999999999999289, 3.065181147996828948 ) ) ;
#2376=VERTEX_POINT ( 'NONE', #295 ) ;
#2381=VECTOR ( 'NONE', #9273, 1000.000000000000114 ) ;
#2388=CARTESIAN_POINT ( 'NONE',  ( -3.339929591309179990, 59.80724097760847968, 34.22175998453048607 ) ) ;
#2390=CARTESIAN_POINT ( 'NONE',  ( -38.00000000000000711, 39.99999999999999289, -3.980288726281173287E-13 ) ) ;
#2391=VECTOR ( 'NONE', #7363, 1000.000000000000000 ) ;
#2392=CARTESIAN_POINT ( 'NONE',  ( 6.597235312685898911, 59.03111057313396515, -35.34929737147491835 ) ) ;
#2397=DIRECTION ( 'NONE',  ( -0.000000000000000000, -1.000000000000000000, -0.000000000000000000 ) ) ;
#2402=CARTESIAN_POINT ( 'NONE',  ( 4.000000000000008882, 0.000000000000000000, 29.00000000000000355 ) ) ;
#2406=DIRECTION ( 'NONE',  ( 1.047444401652940795E-14, 0.000000000000000000, -1.000000000000000000 ) ) ;
#2408=VERTEX_POINT ( 'NONE', #1761 ) ;
#2411=DIRECTION ( 'NONE',  ( 0.000000000000000000, 0.000000000000000000, -1.000000000000000000 ) ) ;
#2412=DIRECTION ( 'NONE',  ( 0.000000000000000000, 0.000000000000000000, -1.000000000000000000 ) ) ;
#2413=DIRECTION ( 'NONE',  ( 0.000000000000000000, 0.000000000000000000, -1.000000000000000000 ) ) ;
#2414=ORIENTED_EDGE ( 'NONE', *, *, #2084, .T. ) ;
#2420=ORIENTED_EDGE ( 'NONE', *, *, #4308, .F. ) ;
#2422=CARTESIAN_POINT ( 'NONE',  ( 0.000000000000000000, 59.99999999999999289, 0.000000000000000000 ) ) ;
#2427=EDGE_CURVE ( 'NONE', #9170, #3565, #4334, .T. ) ;
#2428=CARTESIAN_POINT ( 'NONE',  ( 0.000000000000000000, 39.99999999999999289, 0.000000000000000000 ) ) ;
#2429=AXIS2_PLACEMENT_3D ( 'NONE', #3061, #6080, #1488 ) ;
#2431=EDGE_LOOP ( 'NONE', ( #7002, #7017, #9351, #1046, #3990, #9415 ) ) ;
#2435=VECTOR ( 'NONE', #8326, 999.9999999999998863 ) ;
#2437=CARTESIAN_POINT ( 'NONE',  ( 9.815840903884561541, 59.99999999999999289, -28.34870838944214100 ) ) ;
#2438=CARTESIAN_POINT ( 'NONE',  ( 3.055999436386200419, 59.99999999999998579, -33.03613408327221634 ) ) ;
#2440=CARTESIAN_POINT ( 'NONE',  ( -28.33333333333344939, 39.99999999999999289, 9.860132971832396009 ) ) ;
#2459=ORIENTED_EDGE ( 'NONE', *, *, #690, .F. ) ;
#2462=EDGE_LOOP ( 'NONE', ( #5183, #8086, #2663, #1323 ) ) ;
#2466=DIRECTION ( 'NONE',  ( 0.9449569463147371451, -0.000000000000000000, 0.3271946967961539832 ) ) ;
#2469=CARTESIAN_POINT ( 'NONE',  ( -34.16461100076188018, 59.56421283147439283, -7.812829873186591279 ) ) ;
#2475=DIRECTION ( 'NONE',  ( 0.000000000000000000, 0.000000000000000000, 1.000000000000000000 ) ) ;
#2479=DIRECTION ( 'NONE',  ( 0.6195972517514871658, 0.000000000000000000, 0.7849198975831892522 ) ) ;
#2480=ORIENTED_EDGE ( 'NONE', *, *, #8731, .F. ) ;
#2482=CARTESIAN_POINT ( 'NONE',  ( 4.249163891373067159, 59.35847319192267690, -35.19820543205469221 ) ) ;
#2486=EDGE_CURVE ( 'NONE', #5205, #3216, #8439, .T. ) ;
#2490=DIRECTION ( 'NONE',  ( 0.9444444444444403119, 0.000000000000000000, -0.3286710990611015903 ) ) ;
#2493=DIRECTION ( 'NONE',  ( 0.000000000000000000, 0.000000000000000000, 1.000000000000000000 ) ) ;
#2501=DIRECTION ( 'NONE',  ( -0.7849198975831888081, 0.000000000000000000, 0.6195972517514876099 ) ) ;
#2503=DIRECTION ( 'NONE',  ( 0.000000000000000000, 1.000000000000000000, 0.000000000000000000 ) ) ;
#2509=CARTESIAN_POINT ( 'NONE',  ( 4.000000000000001776, 0.000000000000000000, -24.67792535850613334 ) ) ;
#2511=CIRCLE ( 'NONE', #333, 2.499999999999998668 ) ;
#2513=CARTESIAN_POINT ( 'NONE',  ( -35.56420151578587507, 58.98289357006406419, -5.732470078048709894 ) ) ;
#2515=CARTESIAN_POINT ( 'NONE',  ( 28.33333333333337833, 59.99999999999999289, -9.860132971832594961 ) ) ;
#2517=VERTEX_POINT ( 'NONE', #9519 ) ;
#2525=LINE ( 'NONE', #6433, #951 ) ;
#2527=ORIENTED_EDGE ( 'NONE', *, *, #9495, .F. ) ;
#2529=CARTESIAN_POINT ( 'NONE',  ( 5.775154784098243788, 58.97791112757358434, -35.56426808734907752 ) ) ;
#2530=CARTESIAN_POINT ( 'NONE',  ( -7.848671329280705322, 59.99999999999999289, 32.05305536707737701 ) ) ;
#2543=ORIENTED_EDGE ( 'NONE', *, *, #1544, .F. ) ;
#2547=PLANE ( 'NONE',  #4468 ) ;
#2548=DIRECTION ( 'NONE',  ( 0.000000000000000000, 0.000000000000000000, 1.000000000000000000 ) ) ;
#2549=EDGE_CURVE ( 'NONE', #6432, #279, #8686, .T. ) ;
#2551=CIRCLE ( 'NONE', #1627, 5.000000000000000000 ) ;
#2552=CARTESIAN_POINT ( 'NONE',  ( -24.67792535850613334, 28.99999999999997158, -3.999999999999997335 ) ) ;
#2555=ORIENTED_EDGE ( 'NONE', *, *, #2746, .T. ) ;
#2556=CARTESIAN_POINT ( 'NONE',  ( 32.21437568466744494, 59.99999999999997868, 7.920020133197005485 ) ) ;
#2557=CARTESIAN_POINT ( 'NONE',  ( 0.000000000000000000, 59.99999999999999289, 0.000000000000000000 ) ) ;
#2560=ADVANCED_FACE ( 'NONE', ( #5715 ), #4978, .T. ) ;
#2562=EDGE_CURVE ( 'NONE', #5689, #1692, #2100, .T. ) ;
#2566=DIRECTION ( 'NONE',  ( 0.000000000000000000, 1.000000000000000000, 0.000000000000000000 ) ) ;
#2567=ORIENTED_EDGE ( 'NONE', *, *, #6152, .F. ) ;
#2568=DIRECTION ( 'NONE',  ( 0.9444444444444403119, 0.000000000000000000, -0.3286710990611015903 ) ) ;
#2569=VERTEX_POINT ( 'NONE', #95 ) ;
#2570=ORIENTED_EDGE ( 'NONE', *, *, #3236, .T. ) ;
#2572=DIRECTION ( 'NONE',  ( 0.000000000000000000, 1.000000000000000000, 0.000000000000000000 ) ) ;
#2578=ORIENTED_EDGE ( 'NONE', *, *, #1964, .T. ) ;
#2580=DIRECTION ( 'NONE',  ( -0.000000000000000000, 1.000000000000000000, -0.000000000000000000 ) ) ;
#2587=VECTOR ( 'NONE', #3203, 1000.000000000000000 ) ;
#2589=DIRECTION ( 'NONE',  ( -0.000000000000000000, -1.000000000000000000, -0.000000000000000000 ) ) ;
#2590=ORIENTED_EDGE ( 'NONE', *, *, #4639, .F. ) ;
#2594=AXIS2_PLACEMENT_3D ( 'NONE', #8798, #4454, #2019 ) ;
#2595=ORIENTED_EDGE ( 'NONE', *, *, #4308, .T. ) ;
#2599=ORIENTED_EDGE ( 'NONE', *, *, #2844, .F. ) ;
#2602=FACE_OUTER_BOUND ( 'NONE', #8937, .T. ) ;
#2606=DIRECTION ( 'NONE',  ( 0.000000000000000000, 0.000000000000000000, 1.000000000000000000 ) ) ;
#2608=ORIENTED_EDGE ( 'NONE', *, *, #7889, .T. ) ;
#2609=CARTESIAN_POINT ( 'NONE',  ( 32.71871059427212458, 59.95478203631535052, 8.044358145045418240 ) ) ;
#2611=DIRECTION ( 'NONE',  ( 0.000000000000000000, 1.000000000000000000, 0.000000000000000000 ) ) ;
#2612=ORIENTED_EDGE ( 'NONE', *, *, #6627, .F. ) ;
#2619=EDGE_CURVE ( 'NONE', #4852, #982, #8974, .T. ) ;
#2622=DIRECTION ( 'NONE',  ( -0.000000000000000000, -1.000000000000000000, -0.000000000000000000 ) ) ;
#2624=EDGE_LOOP ( 'NONE', ( #5586, #7289, #3456, #2219, #6564 ) ) ;
#2633=DIRECTION ( 'NONE',  ( -0.9444444444444441977, 0.000000000000000000, 0.3286710990610907657 ) ) ;
#2638=CARTESIAN_POINT ( 'NONE',  ( 4.000000000000007994, 28.99999999999997158, 24.67792535850613334 ) ) ;
#2642=ORIENTED_EDGE ( 'NONE', *, *, #5030, .F. ) ;
#2647=LINE ( 'NONE', #7295, #5444 ) ;
#2648=DIRECTION ( 'NONE',  ( 1.000000000000000000, 0.000000000000000000, -2.168404344971006649E-16 ) ) ;
#2651=DIRECTION ( 'NONE',  ( -0.3271946967961530950, 0.000000000000000000, 0.9449569463147374782 ) ) ;
#2653=CARTESIAN_POINT ( 'NONE',  ( -23.54759692749571087, 59.99999999999999289, 18.58791755254458522 ) ) ;
#2654=DIRECTION ( 'NONE',  ( 0.000000000000000000, 0.000000000000000000, 1.000000000000000000 ) ) ;
#2658=DIRECTION ( 'NONE',  ( 0.000000000000000000, 0.000000000000000000, 1.000000000000000000 ) ) ;
#2662=DIRECTION ( 'NONE',  ( 0.000000000000000000, 1.000000000000000000, 0.000000000000000000 ) ) ;
#2663=ORIENTED_EDGE ( 'NONE', *, *, #2317, .F. ) ;
#2664=DIRECTION ( 'NONE',  ( 0.000000000000000000, 0.000000000000000000, 1.000000000000000000 ) ) ;
#2666=CARTESIAN_POINT ( 'NONE',  ( -29.00000000000000355, 30.00000000000000000, 0.000000000000000000 ) ) ;
#2667=AXIS2_PLACEMENT_3D ( 'NONE', #8873, #5121, #2044 ) ;
#2672=EDGE_CURVE ( 'NONE', #3565, #8321, #3071, .T. ) ;
#2673=DIRECTION ( 'NONE',  ( 0.000000000000000000, 1.000000000000000000, 0.000000000000000000 ) ) ;
#2678=PLANE ( 'NONE',  #2738 ) ;
#2679=EDGE_LOOP ( 'NONE', ( #1600, #9660, #8202, #5625, #143 ) ) ;
#2680=DIRECTION ( 'NONE',  ( 0.6195972517514870548, -0.000000000000000000, 0.7849198975831892522 ) ) ;
#2689=B_SPLINE_CURVE_WITH_KNOTS ( 'NONE', 3,
 ( #5810, #5989, #6589, #6632 ),
 .UNSPECIFIED., .F., .F.,
 ( 4, 4 ),
 ( 0.000000000000000000, 0.001643226871903046308 ),
 .UNSPECIFIED. ) ;
#2690=ORIENTED_EDGE ( 'NONE', *, *, #7129, .T. ) ;
#2691=LINE ( 'NONE', #2094, #6253 ) ;
#2696=CARTESIAN_POINT ( 'NONE',  ( 0.000000000000000000, 30.00000000000000000, 0.000000000000000000 ) ) ;
#2697=CARTESIAN_POINT ( 'NONE',  ( 0.000000000000000000, 59.99999999999999289, 0.000000000000000000 ) ) ;
#2702=ADVANCED_FACE ( 'NONE', ( #2147 ), #8184, .F. ) ;
#2703=ORIENTED_EDGE ( 'NONE', *, *, #9215, .T. ) ;
#2706=VECTOR ( 'NONE', #5501, 1000.000000000000000 ) ;
#2709=DIRECTION ( 'NONE',  ( -0.000000000000000000, -1.000000000000000000, -0.000000000000000000 ) ) ;
#2717=CARTESIAN_POINT ( 'NONE',  ( 35.29563341415538247, 59.05475394944627965, 6.702038549863912564 ) ) ;
#2721=VECTOR ( 'NONE', #4719, 1000.000000000000000 ) ;
#2725=AXIS2_PLACEMENT_3D ( 'NONE', #3625, #7877, #3686 ) ;
#2726=ORIENTED_EDGE ( 'NONE', *, *, #4275, .T. ) ;
#2729=DIRECTION ( 'NONE',  ( 1.000000000000000000, 0.000000000000000000, -1.084202172485503448E-16 ) ) ;
#2730=ORIENTED_EDGE ( 'NONE', *, *, #6913, .T. ) ;
#2732=CARTESIAN_POINT ( 'NONE',  ( 0.000000000000000000, 28.99999999999997158, -29.00000000000000355 ) ) ;
#2733=ADVANCED_FACE ( 'NONE', ( #5596 ), #9454, .T. ) ;
#2736=DIRECTION ( 'NONE',  ( 0.000000000000000000, 0.000000000000000000, 1.000000000000000000 ) ) ;
#2738=AXIS2_PLACEMENT_3D ( 'NONE', #529, #6672, #8121 ) ;
#2740=VECTOR ( 'NONE', #712, 1000.000000000000000 ) ;
#2741=ADVANCED_FACE ( 'NONE', ( #3369 ), #4023, .F. ) ;
#2743=AXIS2_PLACEMENT_3D ( 'NONE', #9717, #5127, #1514 ) ;
#2746=EDGE_CURVE ( 'NONE', #8510, #3565, #8563, .T. ) ;
#2750=PLANE ( 'NONE',  #8590 ) ;
#2754=AXIS2_PLACEMENT_3D ( 'NONE', #1830, #3256, #355 ) ;
#2755=CIRCLE ( 'NONE', #3242, 2.500000000000002220 ) ;
#2757=DIRECTION ( 'NONE',  ( -1.084202172485503325E-16, 0.000000000000000000, -1.000000000000000000 ) ) ;
#2760=CARTESIAN_POINT ( 'NONE',  ( 0.000000000000000000, 54.99999999999999289, 0.000000000000000000 ) ) ;
#2761=VECTOR ( 'NONE', #1383, 1000.000000000000000 ) ;
#2768=FACE_OUTER_BOUND ( 'NONE', #1470, .T. ) ;
#2772=AXIS2_PLACEMENT_3D ( 'NONE', #7906, #1824, #6410 ) ;
#2774=DIRECTION ( 'NONE',  ( -0.000000000000000000, -1.000000000000000000, -0.000000000000000000 ) ) ;
#2775=ORIENTED_EDGE ( 'NONE', *, *, #4415, .T. ) ;
#2779=LINE ( 'NONE', #8809, #998 ) ;
#2782=ORIENTED_EDGE ( 'NONE', *, *, #9508, .F. ) ;
#2784=DIRECTION ( 'NONE',  ( 0.000000000000000000, 0.000000000000000000, 1.000000000000000000 ) ) ;
#2787=DIRECTION ( 'NONE',  ( 8.659560562354904508E-17, -0.7071067811865500152, 0.7071067811865451302 ) ) ;
#2790=DIRECTION ( 'NONE',  ( 0.000000000000000000, 1.000000000000000000, 0.000000000000000000 ) ) ;
#2792=VERTEX_POINT ( 'NONE', #9350 ) ;
#2793=CARTESIAN_POINT ( 'NONE',  ( 35.88888888888889284, 39.99999999999999289, -12.48950176432140502 ) ) ;
#2796=EDGE_CURVE ( 'NONE', #2792, #7616, #6858, .T. ) ;
#2798=CARTESIAN_POINT ( 'NONE',  ( -5.000000000000006217, 30.00000000000000000, 0.000000000000000000 ) ) ;
#2801=ORIENTED_EDGE ( 'NONE', *, *, #6425, .T. ) ;
#2804=EDGE_LOOP ( 'NONE', ( #9256, #826, #6072, #4131 ) ) ;
#2808=EDGE_CURVE ( 'NONE', #9409, #7344, #9396, .T. ) ;
#2811=ORIENTED_EDGE ( 'NONE', *, *, #1877, .T. ) ;
#2815=CARTESIAN_POINT ( 'NONE',  ( 35.42756555166880617, 59.00049740791308039, 6.394654627632705868 ) ) ;
#2816=ORIENTED_EDGE ( 'NONE', *, *, #9461, .T. ) ;
#2817=DIRECTION ( 'NONE',  ( -0.000000000000000000, -1.000000000000000000, -0.000000000000000000 ) ) ;
#2818=VERTEX_POINT ( 'NONE', #9302 ) ;
#2824=ORIENTED_EDGE ( 'NONE', *, *, #5393, .F. ) ;
#2829=CARTESIAN_POINT ( 'NONE',  ( 0.000000000000000000, 59.99999999999999289, 0.000000000000000000 ) ) ;
#2830=DIRECTION ( 'NONE',  ( 0.000000000000000000, 0.000000000000000000, 1.000000000000000000 ) ) ;
#2832=EDGE_CURVE ( 'NONE', #8061, #7838, #6276, .T. ) ;
#2835=CARTESIAN_POINT ( 'NONE',  ( 4.000000000000001776, 28.99999999999997158, -24.67792535850613334 ) ) ;
#2836=ORIENTED_EDGE ( 'NONE', *, *, #7330, .F. ) ;
#2838=VECTOR ( 'NONE', #1024, 1000.000000000000000 ) ;
#2843=( GEOMETRIC_REPRESENTATION_CONTEXT ( 3 ) GLOBAL_UNCERTAINTY_ASSIGNED_CONTEXT ( ( #8322 ) ) GLOBAL_UNIT_ASSIGNED_CONTEXT ( ( #5849, #8867, #1501 ) ) REPRESENTATION_CONTEXT ( 'NONE', 'WORKASPACE' ) );
#2844=EDGE_CURVE ( 'NONE', #5104, #1017, #7118, .T. ) ;
#2845=CARTESIAN_POINT ( 'NONE',  ( 5.000000000000003553, 30.00000000000000000, -1.084202172485504040E-15 ) ) ;
#2849=LINE ( 'NONE', #8887, #5725 ) ;
#2851=EDGE_CURVE ( 'NONE', #1692, #5689, #7181, .T. ) ;
#2854=CYLINDRICAL_SURFACE ( 'NONE', #1144, 38.00000000000000711 ) ;
#2859=CIRCLE ( 'NONE', #5712, 2.499999999999998668 ) ;
#2860=ORIENTED_EDGE ( 'NONE', *, *, #6785, .T. ) ;
#2861=DIRECTION ( 'NONE',  ( 0.000000000000000000, 0.000000000000000000, -1.000000000000000000 ) ) ;
#2862=EDGE_CURVE ( 'NONE', #8986, #9386, #8944, .T. ) ;
#2863=CARTESIAN_POINT ( 'NONE',  ( -3.999999999999999112, 28.99999999999997158, 24.67792535850613334 ) ) ;
#2865=EDGE_CURVE ( 'NONE', #1692, #5147, #7265, .T. ) ;
#2866=ORIENTED_EDGE ( 'NONE', *, *, #3154, .T. ) ;
#2871=VECTOR ( 'NONE', #7541, 1000.000000000000000 ) ;
#2876=DIRECTION ( 'NONE',  ( 1.000000000000000000, -0.000000000000000000, 0.000000000000000000 ) ) ;
#2879=DIRECTION ( 'NONE',  ( 0.000000000000000000, 0.000000000000000000, 1.000000000000000000 ) ) ;
#2881=FACE_OUTER_BOUND ( 'NONE', #8106, .T. ) ;
#2883=CARTESIAN_POINT ( 'NONE',  ( 25.51470164434615029, 30.00000000000000000, 5.000000000000000888 ) ) ;
#2885=PLANE ( 'NONE',  #744 ) ;
#2894=DIRECTION ( 'NONE',  ( 0.000000000000000000, 1.000000000000000000, 0.000000000000000000 ) ) ;
#2896=ORIENTED_EDGE ( 'NONE', *, *, #8248, .T. ) ;
#2905=SHAPE_DEFINITION_REPRESENTATION ( #6219, #551 ) ;
#2908=VERTEX_POINT ( 'NONE', #8161 ) ;
#2909=CARTESIAN_POINT ( 'NONE',  ( -35.05384365671854852, 59.44855477671178079, -4.040090201280811755 ) ) ;
#2911=CARTESIAN_POINT ( 'NONE',  ( 34.33638591132956464, 59.77059716828893698, 3.404146005973824440 ) ) ;
#2914=VERTEX_POINT ( 'NONE', #516 ) ;
#2918=VECTOR ( 'NONE', #8755, 1000.000000000000000 ) ;
#2922=DIRECTION ( 'NONE',  ( 0.000000000000000000, 1.000000000000000000, 0.000000000000000000 ) ) ;
#2923=EDGE_CURVE ( 'NONE', #8994, #5845, #8016, .T. ) ;
#2924=EDGE_CURVE ( 'NONE', #2517, #1478, #7372, .T. ) ;
#2927=AXIS2_PLACEMENT_3D ( 'NONE', #6664, #9688, #3334 ) ;
#2930=EDGE_LOOP ( 'NONE', ( #2155, #2279, #2082, #5887 ) ) ;
#2931=CARTESIAN_POINT ( 'NONE',  ( 0.000000000000000000, 38.99999999999993605, 0.000000000000000000 ) ) ;
#2934=DIRECTION ( 'NONE',  ( 0.000000000000000000, 0.000000000000000000, 1.000000000000000000 ) ) ;
#2939=DIRECTION ( 'NONE',  ( -6.982962677686269077E-15, 0.000000000000000000, 1.000000000000000000 ) ) ;
#2943=CIRCLE ( 'NONE', #8475, 17.99999999999999645 ) ;
#2945=EDGE_CURVE ( 'NONE', #294, #3288, #7172, .T. ) ;
#2948=ADVANCED_FACE ( 'NONE', ( #5197 ), #5154, .T. ) ;
#2952=ORIENTED_EDGE ( 'NONE', *, *, #4051, .T. ) ;
#2955=ORIENTED_EDGE ( 'NONE', *, *, #3964, .T. ) ;
#2960=CARTESIAN_POINT ( 'NONE',  ( -25.51470164434615029, 30.00000000000000000, -4.999999999999997335 ) ) ;
#2963=ORIENTED_EDGE ( 'NONE', *, *, #6261, .F. ) ;
#2964=CARTESIAN_POINT ( 'NONE',  ( 5.562309845534588959, 49.99999999999999289, -33.06426808735054124 ) ) ;
#2965=VERTEX_POINT ( 'NONE', #5050 ) ;
#2968=CARTESIAN_POINT ( 'NONE',  ( -29.00000000000000355, 28.99999999999997158, 4.000000000000010658 ) ) ;
#2969=EDGE_CURVE ( 'NONE', #5003, #5845, #4665, .T. ) ;
#2972=DIRECTION ( 'NONE',  ( 0.000000000000000000, 0.000000000000000000, 1.000000000000000000 ) ) ;
#2978=CARTESIAN_POINT ( 'NONE',  ( 0.000000000000000000, 0.000000000000000000, 0.000000000000000000 ) ) ;
#2979=CARTESIAN_POINT ( 'NONE',  ( -28.34870838944214455, 39.99999999999999289, -9.815840903884556212 ) ) ;
#2980=AXIS2_PLACEMENT_3D ( 'NONE', #1125, #7288, #7138 ) ;
#2982=CARTESIAN_POINT ( 'NONE',  ( 4.665243217607700998, 29.66524321760768501, -25.23917843705063646 ) ) ;
#2984=ORIENTED_EDGE ( 'NONE', *, *, #1550, .F. ) ;
#2987=EDGE_CURVE ( 'NONE', #5863, #9011, #127, .T. ) ;
#2990=EDGE_CURVE ( 'NONE', #9346, #7747, #2207, .T. ) ;
#2991=EDGE_CURVE ( 'NONE', #8562, #4542, #685, .T. ) ;
#2994=ORIENTED_EDGE ( 'NONE', *, *, #2486, .F. ) ;
#3007=DIRECTION ( 'NONE',  ( -0.000000000000000000, -1.000000000000000000, -0.000000000000000000 ) ) ;
#3013=CARTESIAN_POINT ( 'NONE',  ( 29.00000000000000355, 0.000000000000000000, -4.000000000000007105 ) ) ;
#3017=CARTESIAN_POINT ( 'NONE',  ( -7.548108395552116434, 59.38382381638699314, 34.59619211116746129 ) ) ;
#3018=ORIENTED_EDGE ( 'NONE', *, *, #5478, .T. ) ;
#3019=VERTEX_POINT ( 'NONE', #8459 ) ;
#3020=CARTESIAN_POINT ( 'NONE',  ( 0.000000000000000000, 38.99999999999993605, 17.99999999999999645 ) ) ;
#3023=VECTOR ( 'NONE', #7045, 1000.000000000000000 ) ;
#3027=VERTEX_POINT ( 'NONE', #3862 ) ;
#3028=CYLINDRICAL_SURFACE ( 'NONE', #1111, 17.99999999999999645 ) ;
#3037=LINE ( 'NONE', #5272, #715 ) ;
#3039=EDGE_CURVE ( 'NONE', #9639, #22, #9516, .T. ) ;
#3041=CARTESIAN_POINT ( 'NONE',  ( 0.000000000000000000, 39.99999999999999289, 0.000000000000000000 ) ) ;
#3043=DIRECTION ( 'NONE',  ( -0.000000000000000000, -1.000000000000000000, -0.000000000000000000 ) ) ;
#3049=ORIENTED_EDGE ( 'NONE', *, *, #1214, .F. ) ;
#3056=CARTESIAN_POINT ( 'NONE',  ( 25.23917843705063646, 29.66524321760768501, 4.665243217607698334 ) ) ;
#3060=ORIENTED_EDGE ( 'NONE', *, *, #8682, .T. ) ;
#3061=CARTESIAN_POINT ( 'NONE',  ( 33.06426808735054124, 49.99999999999999289, 5.562309845534586294 ) ) ;
#3064=VECTOR ( 'NONE', #7910, 1000.000000000000000 ) ;
#3066=ORIENTED_EDGE ( 'NONE', *, *, #6665, .F. ) ;
#3067=CARTESIAN_POINT ( 'NONE',  ( -7.848671329280705322, 59.99999999999999289, 32.05305536707737701 ) ) ;
#3068=AXIS2_PLACEMENT_3D ( 'NONE', #8399, #9192, #1584 ) ;
#3071=CIRCLE ( 'NONE', #5609, 33.00000000000000000 ) ;
#3072=EDGE_LOOP ( 'NONE', ( #6255, #4777, #5571, #1543 ) ) ;
#3073=TOROIDAL_SURFACE ( 'NONE', #573, 33.00000000000000711, 5.000000000000000000 ) ;
#3076=FACE_OUTER_BOUND ( 'NONE', #8023, .T. ) ;
#3078=CIRCLE ( 'NONE', #5618, 4.999999999999999112 ) ;
#3080=CARTESIAN_POINT ( 'NONE',  ( 12.48950176432140680, 59.99999999999999289, 35.88888888888889284 ) ) ;
#3084=CARTESIAN_POINT ( 'NONE',  ( 0.000000000000000000, 59.99999999999999289, 0.000000000000000000 ) ) ;
#3085=DIRECTION ( 'NONE',  ( 0.000000000000000000, 1.000000000000000000, -0.000000000000000000 ) ) ;
#3090=DIRECTION ( 'NONE',  ( -0.3286710990611143579, -1.387778780781445676E-15, -0.9444444444444359821 ) ) ;
#3093=CARTESIAN_POINT ( 'NONE',  ( 0.000000000000000000, 59.99999999999999289, 0.000000000000000000 ) ) ;
#3095=PLANE ( 'NONE',  #4635 ) ;
#3099=ADVANCED_FACE ( 'NONE', ( #8354 ), #1592, .F. ) ;
#3102=ORIENTED_EDGE ( 'NONE', *, *, #2191, .F. ) ;
#3109=ORIENTED_EDGE ( 'NONE', *, *, #6186, .T. ) ;
#3110=DIRECTION ( 'NONE',  ( 0.5773502691896204020, -0.5773502691896366112, 0.5773502691896204020 ) ) ;
#3111=EDGE_LOOP ( 'NONE', ( #4583, #7158, #2420, #5880, #3513, #1741, #7193, #6576 ) ) ;
#3113=LINE ( 'NONE', #5401, #6214 ) ;
#3118=DIRECTION ( 'NONE',  ( 0.000000000000000000, 1.000000000000000000, 0.000000000000000000 ) ) ;
#3119=ORIENTED_EDGE ( 'NONE', *, *, #8557, .T. ) ;
#3120=ORIENTED_EDGE ( 'NONE', *, *, #2184, .T. ) ;
#3121=DIRECTION ( 'NONE',  ( 2.168404344971006649E-16, -0.000000000000000000, 1.000000000000000000 ) ) ;
#3128=CARTESIAN_POINT ( 'NONE',  ( -4.397412886516822716, 59.29888504437717955, 35.28275170782141146 ) ) ;
#3131=DIRECTION ( 'NONE',  ( 1.000000000000000000, 0.000000000000000000, 3.491481338843137300E-15 ) ) ;
#3138=DIRECTION ( 'NONE',  ( -0.000000000000000000, -1.000000000000000000, -0.000000000000000000 ) ) ;
#3139=CIRCLE ( 'NONE', #2980, 30.00000000000001066 ) ;
#3142=VERTEX_POINT ( 'NONE', #267 ) ;
#3143=LINE ( 'NONE', #2352, #2227 ) ;
#3146=EDGE_CURVE ( 'NONE', #5052, #1776, #5290, .T. ) ;
#3148=AXIS2_PLACEMENT_3D ( 'NONE', #8501, #1730, #4749 ) ;
#3149=CARTESIAN_POINT ( 'NONE',  ( 24.67792535850613334, 28.99999999999997158, 4.000000000000000888 ) ) ;
#3150=EDGE_LOOP ( 'NONE', ( #3322, #2775, #9592, #5647, #7325 ) ) ;
#3153=CARTESIAN_POINT ( 'NONE',  ( -25.23917843705063646, 29.66524321760768501, -4.665243217607696558 ) ) ;
#3154=EDGE_CURVE ( 'NONE', #427, #209, #7973, .T. ) ;
#3155=VECTOR ( 'NONE', #7194, 1000.000000000000000 ) ;
#3156=CARTESIAN_POINT ( 'NONE',  ( 0.000000000000000000, 30.00000000000000000, 0.000000000000000000 ) ) ;
#3162=DIRECTION ( 'NONE',  ( 0.000000000000000000, 0.000000000000000000, 1.000000000000000000 ) ) ;
#3166=EDGE_CURVE ( 'NONE', #2152, #9475, #5637, .T. ) ;
#3167=VERTEX_POINT ( 'NONE', #8699 ) ;
#3168=CARTESIAN_POINT ( 'NONE',  ( -6.597235312685899800, 59.03111057313397225, 35.34929737147492546 ) ) ;
#3170=ORIENTED_EDGE ( 'NONE', *, *, #7689, .T. ) ;
#3174=AXIS2_PLACEMENT_3D ( 'NONE', #8229, #832, #5374 ) ;
#3175=DIRECTION ( 'NONE',  ( -1.084202172485503325E-16, 0.000000000000000000, -1.000000000000000000 ) ) ;
#3177=DIRECTION ( 'NONE',  ( -0.000000000000000000, 1.000000000000000000, -0.000000000000000000 ) ) ;
#3179=CARTESIAN_POINT ( 'NONE',  ( -3.850561375233625849, 59.53730689706332413, 34.89414954626303000 ) ) ;
#3189=EDGE_CURVE ( 'NONE', #7616, #5781, #7757, .T. ) ;
#3191=CARTESIAN_POINT ( 'NONE',  ( -2.304377683636468772E-13, 59.99999999999999289, 33.00000000000000711 ) ) ;
#3196=VECTOR ( 'NONE', #575, 1000.000000000000114 ) ;
#3197=ORIENTED_EDGE ( 'NONE', *, *, #7528, .T. ) ;
#3202=DIRECTION ( 'NONE',  ( 0.9449569463147374782, 1.387778780781445873E-15, 0.3271946967961528729 ) ) ;
#3203=DIRECTION ( 'NONE',  ( 0.7849198975831889191, -0.000000000000000000, -0.6195972517514874989 ) ) ;
#3204=VERTEX_POINT ( 'NONE', #6266 ) ;
#3211=AXIS2_PLACEMENT_3D ( 'NONE', #757, #6127, #2368 ) ;
#3216=VERTEX_POINT ( 'NONE', #4110 ) ;
#3218=ORIENTED_EDGE ( 'NONE', *, *, #7886, .F. ) ;
#3220=EDGE_CURVE ( 'NONE', #7752, #504, #307, .T. ) ;
#3223=EDGE_CURVE ( 'NONE', #9229, #8986, #1503, .T. ) ;
#3227=CARTESIAN_POINT ( 'NONE',  ( -3.619905045646665709, 59.65318172148985099, 34.64718077370495308 ) ) ;
#3231=LINE ( 'NONE', #6245, #5467 ) ;
#3232=DIRECTION ( 'NONE',  ( 1.000000000000000000, 0.000000000000000000, -2.168404344971006649E-16 ) ) ;
#3235=VERTEX_POINT ( 'NONE', #8598 ) ;
#3236=EDGE_CURVE ( 'NONE', #3019, #3425, #7956, .T. ) ;
#3239=AXIS2_PLACEMENT_3D ( 'NONE', #2422, #135, #717 ) ;
#3240=EDGE_CURVE ( 'NONE', #9574, #7738, #6850, .T. ) ;
#3241=VECTOR ( 'NONE', #7440, 1000.000000000000000 ) ;
#3242=AXIS2_PLACEMENT_3D ( 'NONE', #5106, #5159, #6718 ) ;
#3248=CARTESIAN_POINT ( 'NONE',  ( 5.562309845534588959, 49.99999999999999289, -35.56426808735054834 ) ) ;
#3251=LINE ( 'NONE', #5676, #1673 ) ;
#3253=PLANE ( 'NONE',  #1674 ) ;
#3256=DIRECTION ( 'NONE',  ( 0.000000000000000000, 1.000000000000000000, 0.000000000000000000 ) ) ;
#3266=ORIENTED_EDGE ( 'NONE', *, *, #2191, .T. ) ;
#3267=ORIENTED_EDGE ( 'NONE', *, *, #5478, .F. ) ;
#3270=EDGE_CURVE ( 'NONE', #7710, #5104, #9440, .T. ) ;
#3272=ORIENTED_EDGE ( 'NONE', *, *, #4797, .F. ) ;
#3274=EDGE_CURVE ( 'NONE', #3464, #7275, #8124, .T. ) ;
#3277=EDGE_CURVE ( 'NONE', #8953, #9301, #3601, .T. ) ;
#3279=DIRECTION ( 'NONE',  ( 0.000000000000000000, -0.000000000000000000, 1.000000000000000000 ) ) ;
#3281=CARTESIAN_POINT ( 'NONE',  ( 0.000000000000000000, 38.99999999999993605, 17.99999999999999645 ) ) ;
#3283=CARTESIAN_POINT ( 'NONE',  ( -9.815840903884557989, 39.99999999999999289, 28.34870838944214455 ) ) ;
#3286=AXIS2_PLACEMENT_3D ( 'NONE', #4235, #4326, #4919 ) ;
#3288=VERTEX_POINT ( 'NONE', #4210 ) ;
#3289=DIRECTION ( 'NONE',  ( -0.3271946967961528174, 0.000000000000000000, 0.9449569463147374782 ) ) ;
#3291=EDGE_CURVE ( 'NONE', #4557, #179, #877, .T. ) ;
#3294=CARTESIAN_POINT ( 'NONE',  ( 0.000000000000000000, 54.99999999999999289, 0.000000000000000000 ) ) ;
#3297=FACE_OUTER_BOUND ( 'NONE', #3450, .T. ) ;
#3299=CIRCLE ( 'NONE', #3722, 2.500000000000002220 ) ;
#3303=PLANE ( 'NONE',  #5124 ) ;
#3304=ORIENTED_EDGE ( 'NONE', *, *, #1124, .F. ) ;
#3307=DIRECTION ( 'NONE',  ( 0.000000000000000000, 0.000000000000000000, -1.000000000000000000 ) ) ;
#3308=ORIENTED_EDGE ( 'NONE', *, *, #9495, .T. ) ;
#3319=EDGE_LOOP ( 'NONE', ( #1390, #3514, #17, #9431, #1007, #7552 ) ) ;
#3320=CARTESIAN_POINT ( 'NONE',  ( 0.000000000000000000, 39.99999999999999289, 0.000000000000000000 ) ) ;
#3322=ORIENTED_EDGE ( 'NONE', *, *, #9330, .F. ) ;
#3328=FACE_OUTER_BOUND ( 'NONE', #711, .T. ) ;
#3334=DIRECTION ( 'NONE',  ( 0.000000000000000000, 0.000000000000000000, -1.000000000000000000 ) ) ;
#3337=CARTESIAN_POINT ( 'NONE',  ( -30.00000000000001066, 39.99999999999999289, -3.252551416882082410E-13 ) ) ;
#3338=LINE ( 'NONE', #3531, #8751 ) ;
#3344=FACE_OUTER_BOUND ( 'NONE', #3319, .T. ) ;
#3345=DIRECTION ( 'NONE',  ( 0.000000000000000000, 1.000000000000000000, 0.000000000000000000 ) ) ;
#3348=VECTOR ( 'NONE', #1135, 1000.000000000000000 ) ;
#3349=EDGE_CURVE ( 'NONE', #6218, #22, #4400, .T. ) ;
#3352=EDGE_CURVE ( 'NONE', #2376, #2351, #2849, .T. ) ;
#3356=CARTESIAN_POINT ( 'NONE',  ( 8.673617379884035472E-16, 0.000000000000000000, 4.000000000000004441 ) ) ;
#3359=DIRECTION ( 'NONE',  ( -0.000000000000000000, -1.000000000000000000, -0.000000000000000000 ) ) ;
#3362=CARTESIAN_POINT ( 'NONE',  ( 0.000000000000000000, 54.99999999999999289, 0.000000000000000000 ) ) ;
#3366=ORIENTED_EDGE ( 'NONE', *, *, #6896, .F. ) ;
#3367=DIRECTION ( 'NONE',  ( -0.000000000000000000, -1.000000000000000000, -0.000000000000000000 ) ) ;
#3368=ORIENTED_EDGE ( 'NONE', *, *, #2317, .T. ) ;
#3369=FACE_OUTER_BOUND ( 'NONE', #9359, .T. ) ;
#3371=ORIENTED_EDGE ( 'NONE', *, *, #6047, .T. ) ;
#3385=AXIS2_PLACEMENT_3D ( 'NONE', #3041, #4646, #9670 ) ;
#3388=VECTOR ( 'NONE', #6753, 1000.000000000000227 ) ;
#3389=VECTOR ( 'NONE', #1223, 1000.000000000000000 ) ;
#3392=CARTESIAN_POINT ( 'NONE',  ( -28.34870838944214455, 59.99999999999999289, -9.815840903884556212 ) ) ;
#3402=CIRCLE ( 'NONE', #4203, 2.500000000000002220 ) ;
#3407=CIRCLE ( 'NONE', #4680, 2.500000000000002220 ) ;
#3409=ADVANCED_FACE ( 'NONE', ( #8794 ), #1286, .F. ) ;
#3414=EDGE_CURVE ( 'NONE', #2208, #279, #3645, .T. ) ;
#3421=DIRECTION ( 'NONE',  ( -0.000000000000000000, -1.000000000000000000, -0.000000000000000000 ) ) ;
#3422=ORIENTED_EDGE ( 'NONE', *, *, #592, .F. ) ;
#3425=VERTEX_POINT ( 'NONE', #6003 ) ;
#3426=DIRECTION ( 'NONE',  ( 0.000000000000000000, 0.000000000000000000, 1.000000000000000000 ) ) ;
#3427=ORIENTED_EDGE ( 'NONE', *, *, #9520, .T. ) ;
#3429=EDGE_CURVE ( 'NONE', #2569, #4952, #7604, .T. ) ;
#3436=CARTESIAN_POINT ( 'NONE',  ( -18.58791755254458167, 39.99999999999999289, -23.54759692749571087 ) ) ;
#3438=CARTESIAN_POINT ( 'NONE',  ( 0.000000000000000000, 39.99999999999999289, 0.000000000000000000 ) ) ;
#3439=CARTESIAN_POINT ( 'NONE',  ( 0.000000000000000000, 39.99999999999999289, 0.000000000000000000 ) ) ;
#3441=EDGE_CURVE ( 'NONE', #1074, #2338, #2305, .T. ) ;
#3448=DIRECTION ( 'NONE',  ( -0.000000000000000000, -1.000000000000000000, -0.000000000000000000 ) ) ;
#3449=DIRECTION ( 'NONE',  ( 1.000000000000000000, 0.000000000000000000, -2.168404344971006649E-16 ) ) ;
#3450=EDGE_LOOP ( 'NONE', ( #1917, #1603, #2254, #5038 ) ) ;
#3453=CARTESIAN_POINT ( 'NONE',  ( -3.999999999999999112, 28.99999999999997158, 24.67792535850613334 ) ) ;
#3456=ORIENTED_EDGE ( 'NONE', *, *, #237, .F. ) ;
#3457=DIRECTION ( 'NONE',  ( 0.000000000000000000, 0.000000000000000000, 1.000000000000000000 ) ) ;
#3464=VERTEX_POINT ( 'NONE', #1426 ) ;
#3465=PLANE ( 'NONE',  #9394 ) ;
#3469=ORIENTED_EDGE ( 'NONE', *, *, #1676, .T. ) ;
#3477=EDGE_LOOP ( 'NONE', ( #4100, #7642, #4690, #3972, #2480, #5843, #6028 ) ) ;
#3481=PLANE ( 'NONE',  #4485 ) ;
#3482=CYLINDRICAL_SURFACE ( 'NONE', #1260, 30.00000000000001066 ) ;
#3485=DIRECTION ( 'NONE',  ( 1.000000000000000000, 0.000000000000000000, 0.000000000000000000 ) ) ;
#3487=CARTESIAN_POINT ( 'NONE',  ( -32.71871059427212458, 59.95478203631535052, -8.044358145045414688 ) ) ;
#3491=CARTESIAN_POINT ( 'NONE',  ( 9.860132971832495485, 59.99999999999999289, 28.33333333333341031 ) ) ;
#3494=VECTOR ( 'NONE', #3653, 1000.000000000000000 ) ;
#3502=EDGE_LOOP ( 'NONE', ( #1762, #8256, #8302, #4866, #4523 ) ) ;
#3506=AXIS2_PLACEMENT_3D ( 'NONE', #7407, #555, #3554 ) ;
#3510=DIRECTION ( 'NONE',  ( 0.000000000000000000, 0.000000000000000000, 1.000000000000000000 ) ) ;
#3512=DIRECTION ( 'NONE',  ( 0.3271946967961529840, 0.000000000000000000, -0.9449569463147373671 ) ) ;
#3513=ORIENTED_EDGE ( 'NONE', *, *, #4744, .F. ) ;
#3514=ORIENTED_EDGE ( 'NONE', *, *, #6960, .T. ) ;
#3521=EDGE_LOOP ( 'NONE', ( #3469, #6225, #2034, #3018 ) ) ;
#3522=FACE_OUTER_BOUND ( 'NONE', #5320, .T. ) ;
#3523=ORIENTED_EDGE ( 'NONE', *, *, #3223, .F. ) ;
#3524=DIRECTION ( 'NONE',  ( 0.000000000000000000, 1.000000000000000000, -0.000000000000000000 ) ) ;
#3525=EDGE_CURVE ( 'NONE', #982, #156, #3143, .T. ) ;
#3530=EDGE_CURVE ( 'NONE', #3288, #1017, #1468, .T. ) ;
#3531=CARTESIAN_POINT ( 'NONE',  ( 9.815840903884561541, 59.99999999999999289, -28.34870838944214100 ) ) ;
#3538=DIRECTION ( 'NONE',  ( 0.000000000000000000, 1.000000000000000000, 0.000000000000000000 ) ) ;
#3544=ADVANCED_FACE ( 'NONE', ( #7558 ), #3095, .F. ) ;
#3546=VECTOR ( 'NONE', #3512, 1000.000000000000114 ) ;
#3548=MECHANICAL_DESIGN_GEOMETRIC_PRESENTATION_REPRESENTATION('',(#1026),#6851);
#3550=ORIENTED_EDGE ( 'NONE', *, *, #8177, .T. ) ;
#3551=CARTESIAN_POINT ( 'NONE',  ( 0.000000000000000000, 30.00000000000000000, -29.00000000000000355 ) ) ;
#3554=DIRECTION ( 'NONE',  ( 0.000000000000000000, 0.000000000000000000, -1.000000000000000000 ) ) ;
#3556=ORIENTED_EDGE ( 'NONE', *, *, #5581, .T. ) ;
#3559=VECTOR ( 'NONE', #9335, 1000.000000000000000 ) ;
#3565=VERTEX_POINT ( 'NONE', #3905 ) ;
#3566=DIRECTION ( 'NONE',  ( -0.000000000000000000, -1.000000000000000000, -0.000000000000000000 ) ) ;
#3567=VERTEX_POINT ( 'NONE', #788 ) ;
#3568=CARTESIAN_POINT ( 'NONE',  ( 0.000000000000000000, 39.99999999999999289, 0.000000000000000000 ) ) ;
#3569=ORIENTED_EDGE ( 'NONE', *, *, #509, .F. ) ;
#3572=ORIENTED_EDGE ( 'NONE', *, *, #4388, .F. ) ;
#3574=DIRECTION ( 'NONE',  ( -0.000000000000000000, -1.000000000000000000, -0.000000000000000000 ) ) ;
#3578=LINE ( 'NONE', #9650, #4015 ) ;
#3579=ORIENTED_EDGE ( 'NONE', *, *, #8788, .F. ) ;
#3580=CARTESIAN_POINT ( 'NONE',  ( 29.00000000000000355, 28.99999999999997158, -4.000000000000007105 ) ) ;
#3584=EDGE_CURVE ( 'NONE', #9400, #7616, #6893, .T. ) ;
#3585=LINE ( 'NONE', #4385, #3709 ) ;
#3588=ORIENTED_EDGE ( 'NONE', *, *, #2619, .T. ) ;
#3589=DIRECTION ( 'NONE',  ( 0.000000000000000000, -0.000000000000000000, 1.000000000000000000 ) ) ;
#3596=ADVANCED_FACE ( 'NONE', ( #1816 ), #8882, .T. ) ;
#3601=LINE ( 'NONE', #2012, #404 ) ;
#3603=ORIENTED_EDGE ( 'NONE', *, *, #2865, .T. ) ;
#3604=DIRECTION ( 'NONE',  ( -0.000000000000000000, -1.000000000000000000, -0.000000000000000000 ) ) ;
#3610=CARTESIAN_POINT ( 'NONE',  ( 8.673617379884035472E-16, 28.99999999999997158, 4.000000000000004441 ) ) ;
#3615=ORIENTED_EDGE ( 'NONE', *, *, #3274, .T. ) ;
#3620=VECTOR ( 'NONE', #4382, 1000.000000000000000 ) ;
#3622=FACE_OUTER_BOUND ( 'NONE', #3072, .T. ) ;
#3623=VECTOR ( 'NONE', #2589, 1000.000000000000000 ) ;
#3625=CARTESIAN_POINT ( 'NONE',  ( 0.000000000000000000, 59.99999999999999289, 0.000000000000000000 ) ) ;
#3628=DIRECTION ( 'NONE',  ( 0.7849198975831886971, 0.000000000000000000, -0.6195972517514877209 ) ) ;
#3629=VECTOR ( 'NONE', #142, 1000.000000000000000 ) ;
#3635=CIRCLE ( 'NONE', #645, 38.00000000000000711 ) ;
#3636=DIRECTION ( 'NONE',  ( 1.000000000000000000, 0.000000000000000000, -1.084202172485503448E-16 ) ) ;
#3645=LINE ( 'NONE', #6646, #9040 ) ;
#3651=AXIS2_PLACEMENT_3D ( 'NONE', #7995, #2005, #4981 ) ;
#3653=DIRECTION ( 'NONE',  ( -0.000000000000000000, 1.000000000000000000, -0.000000000000000000 ) ) ;
#3659=CIRCLE ( 'NONE', #6488, 37.99999999999999289 ) ;
#3663=CARTESIAN_POINT ( 'NONE',  ( 34.72826512091049267, 59.61718548957851027, 3.689690490709788051 ) ) ;
#3665=DIRECTION ( 'NONE',  ( 0.000000000000000000, 0.000000000000000000, 1.000000000000000000 ) ) ;
#3670=CARTESIAN_POINT ( 'NONE',  ( -9.860132971832692661, 59.99999999999999289, -28.33333333333334281 ) ) ;
#3679=ADVANCED_FACE ( 'NONE', ( #4840 ), #7795, .F. ) ;
#3681=LINE ( 'NONE', #9172, #9153 ) ;
#3686=DIRECTION ( 'NONE',  ( 0.000000000000000000, 0.000000000000000000, -1.000000000000000000 ) ) ;
#3692=AXIS2_PLACEMENT_3D ( 'NONE', #9418, #2633, #6434 ) ;
#3693=AXIS2_PLACEMENT_3D ( 'NONE', #4596, #7602, #9135 ) ;
#3696=CARTESIAN_POINT ( 'NONE',  ( -29.00000000000000355, 28.99999999999997158, 0.000000000000000000 ) ) ;
#3700=ADVANCED_FACE ( 'NONE', ( #3344 ), #7899, .F. ) ;
#3703=CARTESIAN_POINT ( 'NONE',  ( -23.54469556655647722, 39.99999999999999289, -29.82695610816121956 ) ) ;
#3704=ORIENTED_EDGE ( 'NONE', *, *, #8310, .F. ) ;
#3709=VECTOR ( 'NONE', #4425, 1000.000000000000000 ) ;
#3710=ORIENTED_EDGE ( 'NONE', *, *, #1553, .T. ) ;
#3711=CARTESIAN_POINT ( 'NONE',  ( -24.67792535850613334, 0.000000000000000000, -3.999999999999997335 ) ) ;
#3714=CARTESIAN_POINT ( 'NONE',  ( 35.05384365671854852, 59.44855477671178079, 4.040090201280814419 ) ) ;
#3718=VERTEX_POINT ( 'NONE', #6988 ) ;
#3719=VECTOR ( 'NONE', #1876, 1000.000000000000000 ) ;
#3720=CARTESIAN_POINT ( 'NONE',  ( 0.000000000000000000, 1.000000000000014655, -17.99999999999999645 ) ) ;
#3722=AXIS2_PLACEMENT_3D ( 'NONE', #7165, #2662, #7589 ) ;
#3725=ADVANCED_FACE ( 'NONE', ( #547 ), #8784, .F. ) ;
#3726=CIRCLE ( 'NONE', #7348, 38.00000000000000711 ) ;
#3728=CARTESIAN_POINT ( 'NONE',  ( -7.856683717344203011, 59.59863544270933744, 34.07748394475225950 ) ) ;
#3730=LINE ( 'NONE', #7384, #942 ) ;
#3732=CIRCLE ( 'NONE', #4997, 2.500000000000002220 ) ;
#3734=DIRECTION ( 'NONE',  ( 0.000000000000000000, 0.000000000000000000, 1.000000000000000000 ) ) ;
#3737=DIRECTION ( 'NONE',  ( 0.000000000000000000, 0.000000000000000000, 1.000000000000000000 ) ) ;
#3740=DIRECTION ( 'NONE',  ( 0.000000000000000000, 1.000000000000000000, 0.000000000000000000 ) ) ;
#3741=DIRECTION ( 'NONE',  ( 0.000000000000000000, 0.000000000000000000, 1.000000000000000000 ) ) ;
#3744=CARTESIAN_POINT ( 'NONE',  ( 0.000000000000000000, 59.99999999999999289, 0.000000000000000000 ) ) ;
#3758=CARTESIAN_POINT ( 'NONE',  ( -24.96033808169876878, 29.33187429063046991, -4.331874290630485014 ) ) ;
#3761=VERTEX_POINT ( 'NONE', #8689 ) ;
#3762=CARTESIAN_POINT ( 'NONE',  ( 30.00000000000000711, 59.99999999999999289, 1.047444401652940259E-13 ) ) ;
#3767=DIRECTION ( 'NONE',  ( 0.6195972517514877209, -0.000000000000000000, 0.7849198975831889191 ) ) ;
#3769=CYLINDRICAL_SURFACE ( 'NONE', #3239, 30.00000000000000711 ) ;
#3780=AXIS2_PLACEMENT_3D ( 'NONE', #3156, #3007, #2411 ) ;
#3781=CIRCLE ( 'NONE', #1, 38.00000000000000711 ) ;
#3782=ORIENTED_EDGE ( 'NONE', *, *, #3584, .T. ) ;
#3783=DIRECTION ( 'NONE',  ( 0.000000000000000000, 0.000000000000000000, 1.000000000000000000 ) ) ;
#3794=DIRECTION ( 'NONE',  ( 0.000000000000000000, 1.000000000000000000, 0.000000000000000000 ) ) ;
#3801=ORIENTED_EDGE ( 'NONE', *, *, #538, .T. ) ;
#3805=ORIENTED_EDGE ( 'NONE', *, *, #9701, .T. ) ;
#3815=CYLINDRICAL_SURFACE ( 'NONE', #2429, 2.500000000000002220 ) ;
#3819=CIRCLE ( 'NONE', #7123, 2.500000000000002220 ) ;
#3820=ORIENTED_EDGE ( 'NONE', *, *, #2139, .F. ) ;
#3822=PLANE ( 'NONE',  #4428 ) ;
#3823=ORIENTED_EDGE ( 'NONE', *, *, #6249, .T. ) ;
#3828=CARTESIAN_POINT ( 'NONE',  ( -4.000000000000001776, 30.00000000000000000, 4.336808689942015271E-16 ) ) ;
#3829=EDGE_LOOP ( 'NONE', ( #5113, #7685 ) ) ;
#3830=LINE ( 'NONE', #3080, #3629 ) ;
#3834=CARTESIAN_POINT ( 'NONE',  ( -4.249163891373062718, 59.35847319192267690, 35.19820543205469221 ) ) ;
#3837=DIRECTION ( 'NONE',  ( 1.000000000000000000, 0.000000000000000000, -2.168404344971006649E-16 ) ) ;
#3838=ADVANCED_FACE ( 'NONE', ( #4290 ), #1959, .T. ) ;
#3841=CARTESIAN_POINT ( 'NONE',  ( 28.34870838944214100, 59.99999999999999289, 9.815840903884559765 ) ) ;
#3846=PLANE ( 'NONE',  #1105 ) ;
#3852=ORIENTED_EDGE ( 'NONE', *, *, #4716, .T. ) ;
#3853=DIRECTION ( 'NONE',  ( -0.000000000000000000, -1.000000000000000000, -0.000000000000000000 ) ) ;
#3856=ORIENTED_EDGE ( 'NONE', *, *, #8234, .F. ) ;
#3860=CONICAL_SURFACE ( 'NONE', #4969, 26.00000000000000355, 0.7853981633974346233 ) ;
#3862=CARTESIAN_POINT ( 'NONE',  ( -28.33333333333344584, 39.99999999999999289, 9.860132971832394233 ) ) ;
#3863=EDGE_LOOP ( 'NONE', ( #3954, #7242, #8198, #2782 ) ) ;
#3871=CARTESIAN_POINT ( 'NONE',  ( 0.000000000000000000, 39.99999999999999289, 0.000000000000000000 ) ) ;
#3875=DIRECTION ( 'NONE',  ( 1.084202172485503325E-16, 0.000000000000000000, 1.000000000000000000 ) ) ;
#3878=AXIS2_PLACEMENT_3D ( 'NONE', #8014, #8848, #4264 ) ;
#3883=CARTESIAN_POINT ( 'NONE',  ( 12.43339847825378364, 54.99999999999999289, -35.90836395996003461 ) ) ;
#3885=CIRCLE ( 'NONE', #4522, 4.999999999999997335 ) ;
#3887=VERTEX_POINT ( 'NONE', #2793 ) ;
#3892=CARTESIAN_POINT ( 'NONE',  ( 7.848671329280706210, 59.99999999999999289, -32.05305536707737701 ) ) ;
#3895=CARTESIAN_POINT ( 'NONE',  ( -35.90836395996003461, 59.99999999999999289, -12.43339847825377475 ) ) ;
#3899=CARTESIAN_POINT ( 'NONE',  ( 0.000000000000000000, 59.99999999999999289, 0.000000000000000000 ) ) ;
#3902=ORIENTED_EDGE ( 'NONE', *, *, #6785, .F. ) ;
#3904=ORIENTED_EDGE ( 'NONE', *, *, #5656, .F. ) ;
#3905=CARTESIAN_POINT ( 'NONE',  ( 31.16666666666668917, 59.99999999999999289, -10.84614626901589496 ) ) ;
#3912=LINE ( 'NONE', #745, #6855 ) ;
#3915=ORIENTED_EDGE ( 'NONE', *, *, #1951, .T. ) ;
#3916=CARTESIAN_POINT ( 'NONE',  ( 0.000000000000000000, 54.99999999999999289, 38.00000000000000711 ) ) ;
#3920=ORIENTED_EDGE ( 'NONE', *, *, #8991, .T. ) ;
#3923=APPLICATION_CONTEXT ( 'automotive_design' ) ;
#3926=ORIENTED_EDGE ( 'NONE', *, *, #2969, .T. ) ;
#3927=EDGE_LOOP ( 'NONE', ( #6326, #1585, #598, #8617, #2599 ) ) ;
#3929=CARTESIAN_POINT ( 'NONE',  ( 0.000000000000000000, 30.00000000000000000, 0.000000000000000000 ) ) ;
#3930=B_SPLINE_CURVE_WITH_KNOTS ( 'NONE', 3,
 ( #9128, #7032, #924, #6101, #2482, #9313, #5516, #2340, #9224, #9272, #4726, #6144, #5474, #287, #2438, #9177 ),
 .UNSPECIFIED., .F., .F.,
 ( 4, 2, 2, 2, 2, 2, 2, 4 ),
 ( 0.005084922178573566057, 0.006146119420698880481, 0.006676718041761534224, 0.007207316662824187967, 0.007737915283886840842, 0.008268513904949493717, 0.008799112526012148328, 0.009329711147074801203 ),
 .UNSPECIFIED. ) ;
#3931=ORIENTED_EDGE ( 'NONE', *, *, #5776, .T. ) ;
#3932=CARTESIAN_POINT ( 'NONE',  ( 31.18357922838635687, 59.99999999999999289, 10.79742499427301894 ) ) ;
#3933=DIRECTION ( 'NONE',  ( -0.000000000000000000, -1.000000000000000000, -0.000000000000000000 ) ) ;
#3941=LINE ( 'NONE', #5379, #9067 ) ;
#3943=DIRECTION ( 'NONE',  ( 1.000000000000000000, 0.000000000000000000, -1.084202172485503448E-16 ) ) ;
#3944=AXIS2_PLACEMENT_3D ( 'NONE', #6242, #4232, #2479 ) ;
#3953=FACE_OUTER_BOUND ( 'NONE', #6742, .T. ) ;
#3954=ORIENTED_EDGE ( 'NONE', *, *, #3166, .F. ) ;
#3958=ADVANCED_FACE ( 'NONE', ( #5222 ), #5953, .F. ) ;
#3959=CARTESIAN_POINT ( 'NONE',  ( -10.84614626901599799, 54.99999999999999289, -31.16666666666666785 ) ) ;
#3961=ORIENTED_EDGE ( 'NONE', *, *, #2808, .F. ) ;
#3964=EDGE_CURVE ( 'NONE', #3887, #5003, #9648, .T. ) ;
#3965=EDGE_LOOP ( 'NONE', ( #5811, #1765, #4976, #4606 ) ) ;
#3972=ORIENTED_EDGE ( 'NONE', *, *, #4088, .F. ) ;
#3980=DIRECTION ( 'NONE',  ( 1.000000000000000000, 0.000000000000000000, -1.084202172485503325E-16 ) ) ;
#3983=ORIENTED_EDGE ( 'NONE', *, *, #1246, .T. ) ;
#3985=VECTOR ( 'NONE', #4066, 1000.000000000000000 ) ;
#3987=CARTESIAN_POINT ( 'NONE',  ( 0.000000000000000000, 39.99999999999999289, 0.000000000000000000 ) ) ;
#3990=ORIENTED_EDGE ( 'NONE', *, *, #4375, .T. ) ;
#3992=CIRCLE ( 'NONE', #2079, 30.00000000000001066 ) ;
#3993=AXIS2_PLACEMENT_3D ( 'NONE', #1029, #7855, #1079 ) ;
#3997=LINE ( 'NONE', #1080, #7192 ) ;
#4000=AXIS2_PLACEMENT_3D ( 'NONE', #3392, #3289, #6402 ) ;
#4001=DIRECTION ( 'NONE',  ( -1.533293416683393860E-16, -0.7071067811865376918, -0.7071067811865573427 ) ) ;
#4003=ORIENTED_EDGE ( 'NONE', *, *, #6485, .F. ) ;
#4007=CARTESIAN_POINT ( 'NONE',  ( 4.898587196589413815E-15, 30.99999999999998579, -40.00000000000000711 ) ) ;
#4011=ORIENTED_EDGE ( 'NONE', *, *, #7458, .F. ) ;
#4013=DIRECTION ( 'NONE',  ( -0.000000000000000000, 1.000000000000000000, -0.000000000000000000 ) ) ;
#4014=EDGE_CURVE ( 'NONE', #7168, #1933, #4831, .T. ) ;
#4015=VECTOR ( 'NONE', #6671, 1000.000000000000000 ) ;
#4023=PLANE ( 'NONE',  #8922 ) ;
#4025=ORIENTED_EDGE ( 'NONE', *, *, #4642, .F. ) ;
#4029=ADVANCED_FACE ( 'NONE', ( #971 ), #9183, .T. ) ;
#4030=DIRECTION ( 'NONE',  ( -0.6195972517514871658, -0.000000000000000000, -0.7849198975831892522 ) ) ;
#4031=EDGE_CURVE ( 'NONE', #4621, #4883, #5426, .T. ) ;
#4036=CIRCLE ( 'NONE', #9550, 30.00000000000001066 ) ;
#4038=LINE ( 'NONE', #7075, #1284 ) ;
#4039=CARTESIAN_POINT ( 'NONE',  ( 5.987883466156523227, 58.97190912209828895, -35.53684633323564412 ) ) ;
#4042=CARTESIAN_POINT ( 'NONE',  ( 0.000000000000000000, 28.99999999999997158, 0.000000000000000000 ) ) ;
#4044=VECTOR ( 'NONE', #8658, 1000.000000000000000 ) ;
#4045=CIRCLE ( 'NONE', #5307, 30.00000000000000711 ) ;
#4050=DIRECTION ( 'NONE',  ( -1.000000000000000000, 0.000000000000000000, 2.168404344971006649E-16 ) ) ;
#4051=EDGE_CURVE ( 'NONE', #3027, #294, #192, .T. ) ;
#4055=VECTOR ( 'NONE', #1817, 1000.000000000000000 ) ;
#4057=ORIENTED_EDGE ( 'NONE', *, *, #1902, .T. ) ;
#4062=CARTESIAN_POINT ( 'NONE',  ( 0.000000000000000000, 39.99999999999999289, 0.000000000000000000 ) ) ;
#4064=DIRECTION ( 'NONE',  ( -0.000000000000000000, -1.000000000000000000, -0.000000000000000000 ) ) ;
#4065=VERTEX_POINT ( 'NONE', #7034 ) ;
#4066=DIRECTION ( 'NONE',  ( -0.000000000000000000, 1.000000000000000000, -0.000000000000000000 ) ) ;
#4071=CARTESIAN_POINT ( 'NONE',  ( 0.000000000000000000, 59.99999999999999289, 0.000000000000000000 ) ) ;
#4073=CARTESIAN_POINT ( 'NONE',  ( 34.16461100076188018, 59.56421283147439283, 7.812829873186594831 ) ) ;
#4079=ORIENTED_EDGE ( 'NONE', *, *, #5906, .T. ) ;
#4080=CARTESIAN_POINT ( 'NONE',  ( 0.000000000000000000, 59.99999999999999289, 0.000000000000000000 ) ) ;
#4088=EDGE_CURVE ( 'NONE', #252, #7752, #784, .T. ) ;
#4090=ADVANCED_FACE ( 'NONE', ( #5476 ), #289, .T. ) ;
#4092=VECTOR ( 'NONE', #2680, 1000.000000000000114 ) ;
#4094=DIRECTION ( 'NONE',  ( -3.491481338843134539E-15, 0.000000000000000000, 1.000000000000000000 ) ) ;
#4095=VERTEX_POINT ( 'NONE', #9314 ) ;
#4097=EDGE_LOOP ( 'NONE', ( #1907, #8672, #4303, #5025, #3427 ) ) ;
#4100=ORIENTED_EDGE ( 'NONE', *, *, #7951, .F. ) ;
#4110=CARTESIAN_POINT ( 'NONE',  ( 4.000000000000008882, 28.99999999999997158, 29.00000000000000355 ) ) ;
#4111=VERTEX_POINT ( 'NONE', #2530 ) ;
#4113=ORIENTED_EDGE ( 'NONE', *, *, #8310, .T. ) ;
#4114=CIRCLE ( 'NONE', #3148, 2.500000000000002220 ) ;
#4117=DIRECTION ( 'NONE',  ( 0.000000000000000000, 0.000000000000000000, 1.000000000000000000 ) ) ;
#4118=CARTESIAN_POINT ( 'NONE',  ( 0.000000000000000000, 59.99999999999999289, 0.000000000000000000 ) ) ;
#4122=DIRECTION ( 'NONE',  ( -0.6195972517514871658, -0.000000000000000000, -0.7849198975831892522 ) ) ;
#4131=ORIENTED_EDGE ( 'NONE', *, *, #2180, .T. ) ;
#4134=ORIENTED_EDGE ( 'NONE', *, *, #4576, .T. ) ;
#4137=DIRECTION ( 'NONE',  ( -0.000000000000000000, -1.000000000000000000, -0.000000000000000000 ) ) ;
#4152=CARTESIAN_POINT ( 'NONE',  ( 8.673617379884035472E-16, 28.99999999999997158, 4.000000000000004441 ) ) ;
#4154=EDGE_CURVE ( 'NONE', #8074, #1128, #3781, .T. ) ;
#4157=ADVANCED_FACE ( 'NONE', ( #5517 ), #3482, .F. ) ;
#4159=LINE ( 'NONE', #3356, #3559 ) ;
#4164=DIRECTION ( 'NONE',  ( 0.9444444444444315412, 0.000000000000000000, -0.3286710990611267369 ) ) ;
#4177=DIRECTION ( 'NONE',  ( -0.000000000000000000, -1.000000000000000000, -0.000000000000000000 ) ) ;
#4178=CARTESIAN_POINT ( 'NONE',  ( -24.67792535850613334, 28.99999999999997158, -3.999999999999997335 ) ) ;
#4181=PLANE ( 'NONE',  #3944 ) ;
#4182=PLANE ( 'NONE',  #3692 ) ;
#4185=CARTESIAN_POINT ( 'NONE',  ( -29.00000000000000355, 0.000000000000000000, -0.000000000000000000 ) ) ;
#4186=FACE_BOUND ( 'NONE', #9597, .T. ) ;
#4188=CARTESIAN_POINT ( 'NONE',  ( 0.000000000000000000, 0.000000000000000000, 0.000000000000000000 ) ) ;
#4190=VECTOR ( 'NONE', #6166, 1000.000000000000000 ) ;
#4203=AXIS2_PLACEMENT_3D ( 'NONE', #9004, #662, #1302 ) ;
#4204=EDGE_CURVE ( 'NONE', #4449, #6584, #4236, .T. ) ;
#4210=CARTESIAN_POINT ( 'NONE',  ( -29.82695610816121956, 39.99999999999999289, 23.54469556655648432 ) ) ;
#4213=EDGE_CURVE ( 'NONE', #9687, #9170, #1574, .T. ) ;
#4218=DIRECTION ( 'NONE',  ( 0.000000000000000000, 0.7071067811865376918, -0.7071067811865573427 ) ) ;
#4221=ORIENTED_EDGE ( 'NONE', *, *, #5936, .F. ) ;
#4227=ORIENTED_EDGE ( 'NONE', *, *, #5172, .T. ) ;
#4232=DIRECTION ( 'NONE',  ( -0.7849198975831892522, 0.000000000000000000, 0.6195972517514871658 ) ) ;
#4235=CARTESIAN_POINT ( 'NONE',  ( 0.000000000000000000, 59.99999999999999289, 0.000000000000000000 ) ) ;
#4236=LINE ( 'NONE', #4185, #9154 ) ;
#4238=DIRECTION ( 'NONE',  ( -0.000000000000000000, 1.000000000000000000, -0.000000000000000000 ) ) ;
#4240=ORIENTED_EDGE ( 'NONE', *, *, #4579, .T. ) ;
#4241=FACE_BOUND ( 'NONE', #1294, .T. ) ;
#4246=DIRECTION ( 'NONE',  ( -0.000000000000000000, -1.000000000000000000, -0.000000000000000000 ) ) ;
#4247=LINE ( 'NONE', #5674, #7644 ) ;
#4250=DIRECTION ( 'NONE',  ( -2.168404344971006649E-16, 0.000000000000000000, -1.000000000000000000 ) ) ;
#4256=VECTOR ( 'NONE', #3933, 1000.000000000000000 ) ;
#4263=ORIENTED_EDGE ( 'NONE', *, *, #2084, .F. ) ;
#4264=DIRECTION ( 'NONE',  ( 0.000000000000000000, 0.000000000000000000, 1.000000000000000000 ) ) ;
#4266=ORIENTED_EDGE ( 'NONE', *, *, #5170, .F. ) ;
#4269=CIRCLE ( 'NONE', #5378, 2.499999999999998668 ) ;
#4274=AXIS2_PLACEMENT_3D ( 'NONE', #927, #6838, #8432 ) ;
#4275=EDGE_CURVE ( 'NONE', #742, #5194, #5018, .T. ) ;
#4280=EDGE_LOOP ( 'NONE', ( #5747, #2102, #6895, #7703 ) ) ;
#4282=DIRECTION ( 'NONE',  ( 0.000000000000000000, 0.000000000000000000, -1.000000000000000000 ) ) ;
#4290=FACE_OUTER_BOUND ( 'NONE', #1941, .T. ) ;
#4295=VECTOR ( 'NONE', #8153, 1000.000000000000000 ) ;
#4297=DIRECTION ( 'NONE',  ( -1.000000000000000000, 0.000000000000000000, 1.084202172485503448E-16 ) ) ;
#4299=ORIENTED_EDGE ( 'NONE', *, *, #3277, .F. ) ;
#4303=ORIENTED_EDGE ( 'NONE', *, *, #8261, .T. ) ;
#4304=DIRECTION ( 'NONE',  ( 0.000000000000000000, 0.000000000000000000, 1.000000000000000000 ) ) ;
#4308=EDGE_CURVE ( 'NONE', #6509, #8688, #5365, .T. ) ;
#4310=CARTESIAN_POINT ( 'NONE',  ( 0.000000000000000000, 1.000000000000014655, 17.99999999999999645 ) ) ;
#4311=ORIENTED_EDGE ( 'NONE', *, *, #5070, .F. ) ;
#4314=LINE ( 'NONE', #7316, #7355 ) ;
#4315=ORIENTED_EDGE ( 'NONE', *, *, #8557, .F. ) ;
#4317=AXIS2_PLACEMENT_3D ( 'NONE', #3871, #6870, #4117 ) ;
#4326=DIRECTION ( 'NONE',  ( -0.000000000000000000, -1.000000000000000000, -0.000000000000000000 ) ) ;
#4328=EDGE_CURVE ( 'NONE', #7752, #137, #7084, .T. ) ;
#4334=CIRCLE ( 'NONE', #5746, 5.000000000000001776 ) ;
#4343=ORIENTED_EDGE ( 'NONE', *, *, #6720, .T. ) ;
#4348=AXIS2_PLACEMENT_3D ( 'NONE', #2978, #8271, #9608 ) ;
#4349=VECTOR ( 'NONE', #4854, 1000.000000000000000 ) ;
#4351=AXIS2_PLACEMENT_3D ( 'NONE', #7418, #9636, #655 ) ;
#4353=VECTOR ( 'NONE', #6427, 1000.000000000000000 ) ;
#4355=ORIENTED_EDGE ( 'NONE', *, *, #6309, .T. ) ;
#4359=CARTESIAN_POINT ( 'NONE',  ( 24.67792535850613334, 30.00000000000000000, 4.000000000000000888 ) ) ;
#4367=FACE_OUTER_BOUND ( 'NONE', #9503, .T. ) ;
#4369=DIRECTION ( 'NONE',  ( 0.000000000000000000, 1.000000000000000000, 0.000000000000000000 ) ) ;
#4370=ORIENTED_EDGE ( 'NONE', *, *, #7816, .F. ) ;
#4375=EDGE_CURVE ( 'NONE', #6509, #1980, #1361, .T. ) ;
#4377=CIRCLE ( 'NONE', #8569, 4.999999999999999112 ) ;
#4380=ORIENTED_EDGE ( 'NONE', *, *, #2549, .T. ) ;
#4382=DIRECTION ( 'NONE',  ( 1.000000000000000000, -0.000000000000000000, 1.047444401652940795E-14 ) ) ;
#4385=CARTESIAN_POINT ( 'NONE',  ( -3.999999999999998224, 30.00000000000000000, 29.00000000000000355 ) ) ;
#4388=EDGE_CURVE ( 'NONE', #3204, #294, #3730, .T. ) ;
#4389=ORIENTED_EDGE ( 'NONE', *, *, #2832, .T. ) ;
#4391=FACE_OUTER_BOUND ( 'NONE', #9749, .T. ) ;
#4400=LINE ( 'NONE', #3453, #7463 ) ;
#4405=ORIENTED_EDGE ( 'NONE', *, *, #8307, .F. ) ;
#4407=ORIENTED_EDGE ( 'NONE', *, *, #3429, .T. ) ;
#4410=ORIENTED_EDGE ( 'NONE', *, *, #5825, .F. ) ;
#4412=EDGE_LOOP ( 'NONE', ( #8709, #7700, #5963, #4443 ) ) ;
#4415=EDGE_CURVE ( 'NONE', #179, #1752, #6138, .T. ) ;
#4417=LINE ( 'NONE', #8115, #7937 ) ;
#4420=ORIENTED_EDGE ( 'NONE', *, *, #6549, .F. ) ;
#4422=ORIENTED_EDGE ( 'NONE', *, *, #9701, .F. ) ;
#4423=DIRECTION ( 'NONE',  ( 0.000000000000000000, 0.7071067811865451302, 0.7071067811865500152 ) ) ;
#4424=CARTESIAN_POINT ( 'NONE',  ( 0.000000000000000000, 39.99999999999999289, 0.000000000000000000 ) ) ;
#4425=DIRECTION ( 'NONE',  ( -0.000000000000000000, -1.000000000000000000, -0.000000000000000000 ) ) ;
#4426=VECTOR ( 'NONE', #99, 1000.000000000000114 ) ;
#4427=CARTESIAN_POINT ( 'NONE',  ( 4.665243217607707216, 29.66524321760768856, 25.23917843705063646 ) ) ;
#4428=AXIS2_PLACEMENT_3D ( 'NONE', #79, #9061, #4623 ) ;
#4429=ORIENTED_EDGE ( 'NONE', *, *, #8307, .T. ) ;
#4430=EDGE_CURVE ( 'NONE', #7824, #2152, #6133, .T. ) ;
#4431=CARTESIAN_POINT ( 'NONE',  ( -30.00000000000000711, 30.00000000000000000, 0.000000000000000000 ) ) ;
#4432=DIRECTION ( 'NONE',  ( 0.000000000000000000, -0.000000000000000000, 1.000000000000000000 ) ) ;
#4438=EDGE_CURVE ( 'NONE', #5147, #4501, #1402, .T. ) ;
#4443=ORIENTED_EDGE ( 'NONE', *, *, #2844, .T. ) ;
#4444=DIRECTION ( 'NONE',  ( 0.000000000000000000, 0.000000000000000000, 1.000000000000000000 ) ) ;
#4445=DIRECTION ( 'NONE',  ( -1.000000000000000000, 0.000000000000000000, 0.000000000000000000 ) ) ;
#4446=ORIENTED_EDGE ( 'NONE', *, *, #9520, .F. ) ;
#4449=VERTEX_POINT ( 'NONE', #9705 ) ;
#4454=DIRECTION ( 'NONE',  ( 0.000000000000000000, 1.000000000000000000, 0.000000000000000000 ) ) ;
#4455=ORIENTED_EDGE ( 'NONE', *, *, #5775, .F. ) ;
#4458=TOROIDAL_SURFACE ( 'NONE', #7607, 33.00000000000000711, 5.000000000000000000 ) ;
#4461=ORIENTED_EDGE ( 'NONE', *, *, #2184, .F. ) ;
#4463=EDGE_LOOP ( 'NONE', ( #7545, #1272, #3579, #2004 ) ) ;
#4465=ORIENTED_EDGE ( 'NONE', *, *, #8541, .T. ) ;
#4468=AXIS2_PLACEMENT_3D ( 'NONE', #5576, #1823, #3449 ) ;
#4469=DIRECTION ( 'NONE',  ( 0.000000000000000000, 0.000000000000000000, -1.000000000000000000 ) ) ;
#4475=CARTESIAN_POINT ( 'NONE',  ( -30.00000000000001066, 59.99999999999999289, -3.142333204958820777E-13 ) ) ;
#4479=CARTESIAN_POINT ( 'NONE',  ( 5.000000000000002665, 30.00000000000000000, -25.51470164434615029 ) ) ;
#4484=CARTESIAN_POINT ( 'NONE',  ( -4.999999999999998224, 30.00000000000000000, 25.51470164434615029 ) ) ;
#4485=AXIS2_PLACEMENT_3D ( 'NONE', #2732, #6436, #2876 ) ;
#4486=VECTOR ( 'NONE', #2729, 1000.000000000000000 ) ;
#4489=AXIS2_PLACEMENT_3D ( 'NONE', #2697, #5267, #6735 ) ;
#4493=ORIENTED_EDGE ( 'NONE', *, *, #6050, .F. ) ;
#4496=EDGE_CURVE ( 'NONE', #1980, #9059, #6759, .T. ) ;
#4500=CARTESIAN_POINT ( 'NONE',  ( -29.82695610816121956, 54.99999999999999289, 23.54469556655648432 ) ) ;
#4501=VERTEX_POINT ( 'NONE', #7047 ) ;
#4507=CARTESIAN_POINT ( 'NONE',  ( 4.000000000000001776, 0.000000000000000000, -29.00000000000000355 ) ) ;
#4510=EDGE_CURVE ( 'NONE', #8890, #4111, #4114, .T. ) ;
#4512=DIRECTION ( 'NONE',  ( 0.000000000000000000, 0.000000000000000000, 1.000000000000000000 ) ) ;
#4515=AXIS2_PLACEMENT_3D ( 'NONE', #7057, #7961, #1976 ) ;
#4517=AXIS2_PLACEMENT_3D ( 'NONE', #6178, #1697, #7625 ) ;
#4522=AXIS2_PLACEMENT_3D ( 'NONE', #1566, #1754, #3131 ) ;
#4523=ORIENTED_EDGE ( 'NONE', *, *, #8261, .F. ) ;
#4525=EDGE_LOOP ( 'NONE', ( #2247, #9388, #7251, #314 ) ) ;
#4532=PLANE ( 'NONE',  #9196 ) ;
#4533=ADVANCED_FACE ( 'NONE', ( #6310 ), #6924, .F. ) ;
#4535=ORIENTED_EDGE ( 'NONE', *, *, #5013, .T. ) ;
#4536=DIRECTION ( 'NONE',  ( 0.000000000000000000, 1.000000000000000000, 0.000000000000000000 ) ) ;
#4537=CARTESIAN_POINT ( 'NONE',  ( -2.094888803305880518E-13, 59.99999999999999289, 30.00000000000000711 ) ) ;
#4541=DIRECTION ( 'NONE',  ( -0.000000000000000000, -1.000000000000000000, -0.000000000000000000 ) ) ;
#4542=VERTEX_POINT ( 'NONE', #2883 ) ;
#4548=ORIENTED_EDGE ( 'NONE', *, *, #6420, .F. ) ;
#4554=ORIENTED_EDGE ( 'NONE', *, *, #4797, .T. ) ;
#4555=CARTESIAN_POINT ( 'NONE',  ( -28.34870838944214455, 59.99999999999999289, -9.815840903884556212 ) ) ;
#4557=VERTEX_POINT ( 'NONE', #8176 ) ;
#4558=CARTESIAN_POINT ( 'NONE',  ( 9.860132971832495485, 39.99999999999999289, 28.33333333333341031 ) ) ;
#4570=UNCERTAINTY_MEASURE_WITH_UNIT (LENGTH_MEASURE( 1.000000000000000082E-05 ), #2176, 'distance_accuracy_value', 'NONE');
#4576=EDGE_CURVE ( 'NONE', #9368, #2152, #2689, .T. ) ;
#4579=EDGE_CURVE ( 'NONE', #6748, #5855, #1166, .T. ) ;
#4580=ORIENTED_EDGE ( 'NONE', *, *, #74, .T. ) ;
#4581=DIRECTION ( 'NONE',  ( 0.000000000000000000, 0.000000000000000000, 1.000000000000000000 ) ) ;
#4582=DIRECTION ( 'NONE',  ( 0.000000000000000000, 1.000000000000000000, 0.000000000000000000 ) ) ;
#4583=ORIENTED_EDGE ( 'NONE', *, *, #1951, .F. ) ;
#4585=DIRECTION ( 'NONE',  ( 0.000000000000000000, 0.000000000000000000, -1.000000000000000000 ) ) ;
#4587=CARTESIAN_POINT ( 'NONE',  ( 6.397328100368729231, 58.99819947112212759, -35.43017184758411986 ) ) ;
#4592=VECTOR ( 'NONE', #5897, 1000.000000000000000 ) ;
#4594=CARTESIAN_POINT ( 'NONE',  ( 10.84614626901677248, 54.99999999999999289, 31.16666666666639784 ) ) ;
#4596=CARTESIAN_POINT ( 'NONE',  ( 20.44670930779908247, 54.99999999999999289, 25.90235662024525709 ) ) ;
#4600=ADVANCED_FACE ( 'NONE', ( #5949 ), #7486, .T. ) ;
#4604=EDGE_CURVE ( 'NONE', #8554, #3204, #1416, .T. ) ;
#4606=ORIENTED_EDGE ( 'NONE', *, *, #5776, .F. ) ;
#4611=DIRECTION ( 'NONE',  ( 0.000000000000000000, 0.000000000000000000, -1.000000000000000000 ) ) ;
#4613=ORIENTED_EDGE ( 'NONE', *, *, #7886, .T. ) ;
#4617=PLANE ( 'NONE',  #8715 ) ;
#4621=VERTEX_POINT ( 'NONE', #8821 ) ;
#4623=DIRECTION ( 'NONE',  ( -1.000000000000000000, 0.000000000000000000, 1.084202172485503448E-16 ) ) ;
#4627=CIRCLE ( 'NONE', #1149, 19.00000000000005684 ) ;
#4630=DIRECTION ( 'NONE',  ( -0.000000000000000000, -1.000000000000000000, -0.000000000000000000 ) ) ;
#4633=CARTESIAN_POINT ( 'NONE',  ( -32.92587516511807166, 59.99999999999999289, -3.065181147996824507 ) ) ;
#4635=AXIS2_PLACEMENT_3D ( 'NONE', #3696, #7504, #1625 ) ;
#4636=ORIENTED_EDGE ( 'NONE', *, *, #1676, .F. ) ;
#4638=LINE ( 'NONE', #1616, #4990 ) ;
#4639=EDGE_CURVE ( 'NONE', #5003, #4849, #1319, .T. ) ;
#4642=EDGE_CURVE ( 'NONE', #5205, #6457, #6331, .T. ) ;
#4646=DIRECTION ( 'NONE',  ( -0.000000000000000000, -1.000000000000000000, -0.000000000000000000 ) ) ;
#4648=CARTESIAN_POINT ( 'NONE',  ( 20.99999999999999645, 0.000000000000000000, 4.000000000000000888 ) ) ;
#4657=CARTESIAN_POINT ( 'NONE',  ( 5.000000000000002665, 30.00000000000000000, -30.00000000000000711 ) ) ;
#4661=CARTESIAN_POINT ( 'NONE',  ( 0.000000000000000000, 0.000000000000000000, 0.000000000000000000 ) ) ;
#4663=DIRECTION ( 'NONE',  ( 1.000000000000000000, 0.000000000000000000, -2.168404344971006649E-16 ) ) ;
#4665=CIRCLE ( 'NONE', #7009, 37.99999999999999289 ) ;
#4666=VECTOR ( 'NONE', #1317, 1000.000000000000000 ) ;
#4670=ORIENTED_EDGE ( 'NONE', *, *, #8544, .F. ) ;
#4671=CONICAL_SURFACE ( 'NONE', #1196, 17.99999999999999645, 0.7853981633974517207 ) ;
#4672=AXIS2_PLACEMENT_3D ( 'NONE', #40, #6040, #3837 ) ;
#4673=ORIENTED_EDGE ( 'NONE', *, *, #7943, .T. ) ;
#4674=AXIS2_PLACEMENT_3D ( 'NONE', #1564, #8332, #4585 ) ;
#4677=( NAMED_UNIT ( * ) SI_UNIT ( $, .STERADIAN. ) SOLID_ANGLE_UNIT ( ) );
#4680=AXIS2_PLACEMENT_3D ( 'NONE', #8458, #7753, #9382 ) ;
#4681=ORIENTED_EDGE ( 'NONE', *, *, #3349, .F. ) ;
#4682=DIRECTION ( 'NONE',  ( -0.000000000000000000, -1.000000000000000000, -0.000000000000000000 ) ) ;
#4684=DIRECTION ( 'NONE',  ( 0.000000000000000000, 0.000000000000000000, -1.000000000000000000 ) ) ;
#4685=CARTESIAN_POINT ( 'NONE',  ( 7.420105108763668689, 59.31303094616893645, -34.74949143486232828 ) ) ;
#4689=CARTESIAN_POINT ( 'NONE',  ( 29.82695610816121956, 39.99999999999999289, -23.54469556655648077 ) ) ;
#4690=ORIENTED_EDGE ( 'NONE', *, *, #4328, .F. ) ;
#4708=DIRECTION ( 'NONE',  ( -1.000000000000000000, 0.000000000000000000, 0.000000000000000000 ) ) ;
#4710=FACE_OUTER_BOUND ( 'NONE', #6962, .T. ) ;
#4715=ORIENTED_EDGE ( 'NONE', *, *, #3189, .T. ) ;
#4716=EDGE_CURVE ( 'NONE', #137, #6352, #325, .T. ) ;
#4719=DIRECTION ( 'NONE',  ( -0.000000000000000000, -1.000000000000000000, -0.000000000000000000 ) ) ;
#4720=EDGE_CURVE ( 'NONE', #7878, #4449, #7543, .T. ) ;
#4721=ORIENTED_EDGE ( 'NONE', *, *, #983, .F. ) ;
#4725=LINE ( 'NONE', #7733, #6322 ) ;
#4726=CARTESIAN_POINT ( 'NONE',  ( 3.265277612493203918, 59.85134567364465141, -34.06652594440189574 ) ) ;
#4729=DIRECTION ( 'NONE',  ( -0.000000000000000000, -1.000000000000000000, -0.000000000000000000 ) ) ;
#4731=DIRECTION ( 'NONE',  ( 0.000000000000000000, 0.000000000000000000, 1.000000000000000000 ) ) ;
#4733=EDGE_CURVE ( 'NONE', #2965, #2351, #6881, .T. ) ;
#4734=CARTESIAN_POINT ( 'NONE',  ( 24.67792535850613334, 28.99999999999997158, 4.000000000000000888 ) ) ;
#4736=ORIENTED_EDGE ( 'NONE', *, *, #5087, .T. ) ;
#4737=DIRECTION ( 'NONE',  ( 2.168404344971006649E-16, 0.000000000000000000, 1.000000000000000000 ) ) ;
#4739=ORIENTED_EDGE ( 'NONE', *, *, #4733, .T. ) ;
#4744=EDGE_CURVE ( 'NONE', #7534, #880, #1385, .T. ) ;
#4746=AXIS2_PLACEMENT_3D ( 'NONE', #7986, #4238, #8726 ) ;
#4749=DIRECTION ( 'NONE',  ( 0.000000000000000000, 0.000000000000000000, 1.000000000000000000 ) ) ;
#4751=ADVANCED_FACE ( 'NONE', ( #6778 ), #967, .F. ) ;
#4753=VERTEX_POINT ( 'NONE', #3932 ) ;
#4756=DIRECTION ( 'NONE',  ( 0.000000000000000000, 0.000000000000000000, 1.000000000000000000 ) ) ;
#4759=EDGE_CURVE ( 'NONE', #252, #2338, #4269, .T. ) ;
#4764=CARTESIAN_POINT ( 'NONE',  ( -34.92646553026882117, 59.22976218012610161, -7.237999934912877187 ) ) ;
#4766=DIRECTION ( 'NONE',  ( -1.000000000000000000, 0.000000000000000000, 0.000000000000000000 ) ) ;
#4768=ORIENTED_EDGE ( 'NONE', *, *, #5585, .F. ) ;
#4770=EDGE_CURVE ( 'NONE', #1752, #2376, #7588, .T. ) ;
#4771=DIRECTION ( 'NONE',  ( 0.000000000000000000, 0.000000000000000000, 1.000000000000000000 ) ) ;
#4773=CARTESIAN_POINT ( 'NONE',  ( -28.33333333333344939, 59.99999999999999289, 9.860132971832396009 ) ) ;
#4774=ADVANCED_FACE ( 'NONE', ( #9171 ), #3028, .F. ) ;
#4775=ORIENTED_EDGE ( 'NONE', *, *, #7943, .F. ) ;
#4777=ORIENTED_EDGE ( 'NONE', *, *, #8008, .T. ) ;
#4779=AXIS2_PLACEMENT_3D ( 'NONE', #7903, #4001, #2648 ) ;
#4780=CARTESIAN_POINT ( 'NONE',  ( 8.070750150710592763, 59.89221580632705155, -33.08193339022353996 ) ) ;
#4788=VERTEX_POINT ( 'NONE', #2288 ) ;
#4791=CIRCLE ( 'NONE', #542, 5.000000000000001776 ) ;
#4792=VERTEX_POINT ( 'NONE', #9072 ) ;
#4796=DIRECTION ( 'NONE',  ( 1.000000000000000000, -0.000000000000000000, 0.000000000000000000 ) ) ;
#4797=EDGE_CURVE ( 'NONE', #6432, #3019, #5523, .T. ) ;
#4801=ORIENTED_EDGE ( 'NONE', *, *, #1707, .T. ) ;
#4803=CARTESIAN_POINT ( 'NONE',  ( 0.000000000000000000, 59.99999999999999289, 0.000000000000000000 ) ) ;
#4810=EDGE_CURVE ( 'NONE', #1652, #4857, #3830, .T. ) ;
#4811=VECTOR ( 'NONE', #4250, 1000.000000000000000 ) ;
#4813=CARTESIAN_POINT ( 'NONE',  ( -35.56433427405016090, 59.02194934605864063, -5.394111410765020764 ) ) ;
#4815=ORIENTED_EDGE ( 'NONE', *, *, #3039, .F. ) ;
#4816=CARTESIAN_POINT ( 'NONE',  ( -23.54759692749571087, 59.99999999999999289, 18.58791755254458877 ) ) ;
#4829=DIRECTION ( 'NONE',  ( 0.5773502691896204020, -0.5773502691896366112, 0.5773502691896204020 ) ) ;
#4831=LINE ( 'NONE', #8428, #6489 ) ;
#4832=CARTESIAN_POINT ( 'NONE',  ( 0.000000000000000000, 59.99999999999999289, 0.000000000000000000 ) ) ;
#4836=ORIENTED_EDGE ( 'NONE', *, *, #2851, .F. ) ;
#4837=FACE_OUTER_BOUND ( 'NONE', #839, .T. ) ;
#4840=FACE_OUTER_BOUND ( 'NONE', #9219, .T. ) ;
#4841=DIRECTION ( 'NONE',  ( 0.000000000000000000, 1.000000000000000000, 0.000000000000000000 ) ) ;
#4849=VERTEX_POINT ( 'NONE', #5263 ) ;
#4850=DIRECTION ( 'NONE',  ( -0.000000000000000000, -1.000000000000000000, -0.000000000000000000 ) ) ;
#4852=VERTEX_POINT ( 'NONE', #9124 ) ;
#4854=DIRECTION ( 'NONE',  ( -0.000000000000000000, -1.000000000000000000, -0.000000000000000000 ) ) ;
#4855=VERTEX_POINT ( 'NONE', #8275 ) ;
#4857=VERTEX_POINT ( 'NONE', #8671 ) ;
#4864=ADVANCED_FACE ( 'NONE', ( #8718 ), #1014, .T. ) ;
#4866=ORIENTED_EDGE ( 'NONE', *, *, #1461, .T. ) ;
#4868=ORIENTED_EDGE ( 'NONE', *, *, #4604, .T. ) ;
#4876=ADVANCED_FACE ( 'NONE', ( #438 ), #4181, .F. ) ;
#4879=CARTESIAN_POINT ( 'NONE',  ( 28.33333333333337833, 39.99999999999999289, -9.860132971832594961 ) ) ;
#4883=VERTEX_POINT ( 'NONE', #327 ) ;
#4884=CARTESIAN_POINT ( 'NONE',  ( 0.000000000000000000, 54.99999999999999289, 0.000000000000000000 ) ) ;
#4885=DIRECTION ( 'NONE',  ( -0.000000000000000000, -1.000000000000000000, -0.000000000000000000 ) ) ;
#4886=DIRECTION ( 'NONE',  ( 1.000000000000000000, 0.000000000000000000, 0.000000000000000000 ) ) ;
#4887=AXIS2_PLACEMENT_3D ( 'NONE', #5369, #1096, #1561 ) ;
#4890=EDGE_LOOP ( 'NONE', ( #1228, #1176, #5405, #2824, #437, #8243, #3422, #4636, #8369, #7073, #9691, #26, #2590, #3926, #666, #7991, #2543, #8200, #3366, #7841, #4721, #367, #7721, #2195, #6756, #4113, #9326, #370, #5440, #8732, #6415, #3102 ) ) ;
#4891=CARTESIAN_POINT ( 'NONE',  ( -23.54759692749571087, 59.99999999999999289, 18.58791755254458522 ) ) ;
#4894=DIRECTION ( 'NONE',  ( 0.000000000000000000, 0.000000000000000000, 1.000000000000000000 ) ) ;
#4904=VECTOR ( 'NONE', #4541, 1000.000000000000000 ) ;
#4906=DIRECTION ( 'NONE',  ( -0.000000000000000000, -1.000000000000000000, -0.000000000000000000 ) ) ;
#4907=EDGE_LOOP ( 'NONE', ( #1696, #7040, #5496, #7781, #6108 ) ) ;
#4908=DIRECTION ( 'NONE',  ( 0.000000000000000000, 0.000000000000000000, 1.000000000000000000 ) ) ;
#4909=ORIENTED_EDGE ( 'NONE', *, *, #535, .F. ) ;
#4914=VECTOR ( 'NONE', #1069, 1000.000000000000000 ) ;
#4919=DIRECTION ( 'NONE',  ( 0.000000000000000000, 0.000000000000000000, -1.000000000000000000 ) ) ;
#4923=DIRECTION ( 'NONE',  ( 0.000000000000000000, 1.000000000000000000, 0.000000000000000000 ) ) ;
#4926=CIRCLE ( 'NONE', #1922, 38.00000000000000711 ) ;
#4934=ORIENTED_EDGE ( 'NONE', *, *, #2746, .F. ) ;
#4936=LINE ( 'NONE', #2006, #1521 ) ;
#4938=LINE ( 'NONE', #4152, #3023 ) ;
#4944=DIRECTION ( 'NONE',  ( -0.000000000000000000, -0.000000000000000000, 1.000000000000000000 ) ) ;
#4945=DIRECTION ( 'NONE',  ( 0.000000000000000000, 1.000000000000000000, 0.000000000000000000 ) ) ;
#4947=DIRECTION ( 'NONE',  ( -0.3286710990610907657, 0.000000000000000000, -0.9444444444444440867 ) ) ;
#4952=VERTEX_POINT ( 'NONE', #378 ) ;
#4955=CARTESIAN_POINT ( 'NONE',  ( 9.860132971832495485, 59.99999999999999289, 28.33333333333341031 ) ) ;
#4956=ORIENTED_EDGE ( 'NONE', *, *, #7218, .T. ) ;
#4957=ORIENTED_EDGE ( 'NONE', *, *, #8719, .T. ) ;
#4965=ORIENTED_EDGE ( 'NONE', *, *, #352, .F. ) ;
#4967=LINE ( 'NONE', #6483, #311 ) ;
#4969=AXIS2_PLACEMENT_3D ( 'NONE', #2696, #5629, #6407 ) ;
#4971=DIRECTION ( 'NONE',  ( 0.000000000000000000, 0.000000000000000000, 1.000000000000000000 ) ) ;
#4973=EDGE_CURVE ( 'NONE', #8688, #742, #2525, .T. ) ;
#4976=ORIENTED_EDGE ( 'NONE', *, *, #8177, .F. ) ;
#4977=DIRECTION ( 'NONE',  ( -0.6195972517514870548, 0.000000000000000000, -0.7849198975831892522 ) ) ;
#4978=PLANE ( 'NONE',  #4489 ) ;
#4981=DIRECTION ( 'NONE',  ( -1.000000000000000000, 0.000000000000000000, 1.084202172485503448E-16 ) ) ;
#4983=VECTOR ( 'NONE', #7380, 1000.000000000000000 ) ;
#4985=VECTOR ( 'NONE', #522, 1000.000000000000000 ) ;
#4987=EDGE_CURVE ( 'NONE', #880, #6509, #8043, .T. ) ;
#4990=VECTOR ( 'NONE', #8526, 1000.000000000000000 ) ;
#4997=AXIS2_PLACEMENT_3D ( 'NONE', #1380, #4945, #2654 ) ;
#5000=DIRECTION ( 'NONE',  ( 0.000000000000000000, -1.000000000000000000, 0.000000000000000000 ) ) ;
#5003=VERTEX_POINT ( 'NONE', #4689 ) ;
#5004=CARTESIAN_POINT ( 'NONE',  ( -33.06426808735054124, 59.99576382555915899, -3.062309845534580077 ) ) ;
#5006=CARTESIAN_POINT ( 'NONE',  ( 35.54742948121823787, 59.05243086228237104, 5.228649803729175538 ) ) ;
#5013=EDGE_CURVE ( 'NONE', #6355, #6584, #780, .T. ) ;
#5014=ORIENTED_EDGE ( 'NONE', *, *, #4720, .F. ) ;
#5018=LINE ( 'NONE', #5115, #8830 ) ;
#5021=CARTESIAN_POINT ( 'NONE',  ( 29.00000000000000355, 28.99999999999997158, -4.000000000000007105 ) ) ;
#5022=EDGE_LOOP ( 'NONE', ( #3266, #7088, #5312, #4739 ) ) ;
#5023=PLANE ( 'NONE',  #6695 ) ;
#5025=ORIENTED_EDGE ( 'NONE', *, *, #1233, .T. ) ;
#5028=DIRECTION ( 'NONE',  ( -0.9444444444444315412, 0.000000000000000000, 0.3286710990611268479 ) ) ;
#5030=EDGE_CURVE ( 'NONE', #1752, #1969, #3635, .T. ) ;
#5031=FACE_OUTER_BOUND ( 'NONE', #8083, .T. ) ;
#5038=ORIENTED_EDGE ( 'NONE', *, *, #9033, .T. ) ;
#5039=CARTESIAN_POINT ( 'NONE',  ( 33.06426808735054124, 49.99999999999999289, 8.062309845534588959 ) ) ;
#5045=ADVANCED_FACE ( 'NONE', ( #7551 ), #8694, .T. ) ;
#5046=ORIENTED_EDGE ( 'NONE', *, *, #5581, .F. ) ;
#5050=CARTESIAN_POINT ( 'NONE',  ( -2.094888803305880518E-13, 59.99999999999999289, 30.00000000000000711 ) ) ;
#5052=VERTEX_POINT ( 'NONE', #6982 ) ;
#5054=VECTOR ( 'NONE', #921, 1000.000000000000000 ) ;
#5062=CARTESIAN_POINT ( 'NONE',  ( 0.000000000000000000, 39.99999999999999289, 0.000000000000000000 ) ) ;
#5066=AXIS2_PLACEMENT_3D ( 'NONE', #6288, #7846, #7079 ) ;
#5070=EDGE_CURVE ( 'NONE', #2338, #9259, #2511, .T. ) ;
#5074=FACE_OUTER_BOUND ( 'NONE', #8522, .T. ) ;
#5080=CARTESIAN_POINT ( 'NONE',  ( 4.000000000000001776, 30.00000000000000000, 0.000000000000000000 ) ) ;
#5083=DIRECTION ( 'NONE',  ( 0.000000000000000000, 1.000000000000000000, 0.000000000000000000 ) ) ;
#5085=DIRECTION ( 'NONE',  ( -0.000000000000000000, -1.000000000000000000, -0.000000000000000000 ) ) ;
#5087=EDGE_CURVE ( 'NONE', #6014, #4753, #835, .T. ) ;
#5090=FACE_OUTER_BOUND ( 'NONE', #338, .T. ) ;
#5091=CARTESIAN_POINT ( 'NONE',  ( 25.90235662024527485, 59.99999999999999289, -20.44670930779904339 ) ) ;
#5093=VECTOR ( 'NONE', #4030, 1000.000000000000114 ) ;
#5094=VECTOR ( 'NONE', #5384, 1000.000000000000000 ) ;
#5098=CARTESIAN_POINT ( 'NONE',  ( -34.60286690457041914, 59.67177527313210561, -3.585274540811277610 ) ) ;
#5100=CARTESIAN_POINT ( 'NONE',  ( 35.21620900558183820, 59.09151583898437821, 6.845072491844678808 ) ) ;
#5101=ORIENTED_EDGE ( 'NONE', *, *, #201, .F. ) ;
#5104=VERTEX_POINT ( 'NONE', #6888 ) ;
#5106=CARTESIAN_POINT ( 'NONE',  ( -5.562309845534584518, 49.99999999999999289, 33.06426808735054124 ) ) ;
#5107=DIRECTION ( 'NONE',  ( 0.000000000000000000, 0.000000000000000000, 1.000000000000000000 ) ) ;
#5110=ADVANCED_FACE ( 'NONE', ( #5616 ), #5756, .F. ) ;
#5112=DIRECTION ( 'NONE',  ( -0.000000000000000000, -1.000000000000000000, -0.000000000000000000 ) ) ;
#5113=ORIENTED_EDGE ( 'NONE', *, *, #396, .T. ) ;
#5115=CARTESIAN_POINT ( 'NONE',  ( -30.00000000000001066, 39.99999999999999289, -3.142333204958820777E-13 ) ) ;
#5116=DIRECTION ( 'NONE',  ( 0.000000000000000000, 1.000000000000000000, 0.000000000000000000 ) ) ;
#5121=DIRECTION ( 'NONE',  ( -0.000000000000000000, -1.000000000000000000, -0.000000000000000000 ) ) ;
#5123=EDGE_LOOP ( 'NONE', ( #4548, #7216, #8386, #394 ) ) ;
#5124=AXIS2_PLACEMENT_3D ( 'NONE', #6313, #5083, #7204 ) ;
#5125=CARTESIAN_POINT ( 'NONE',  ( -18.58791755254457456, 39.99999999999999289, -23.54759692749571443 ) ) ;
#5127=DIRECTION ( 'NONE',  ( 0.000000000000000000, -1.000000000000000000, 0.000000000000000000 ) ) ;
#5129=DIRECTION ( 'NONE',  ( -0.3271946967961527619, -0.000000000000000000, 0.9449569463147374782 ) ) ;
#5131=AXIS2_PLACEMENT_3D ( 'NONE', #6413, #2503, #5539 ) ;
#5134=VECTOR ( 'NONE', #7562, 1000.000000000000000 ) ;
#5136=PLANE ( 'NONE',  #9697 ) ;
#5137=AXIS2_PLACEMENT_3D ( 'NONE', #2666, #4766, #428 ) ;
#5138=EDGE_CURVE ( 'NONE', #8953, #2569, #7905, .T. ) ;
#5139=ORIENTED_EDGE ( 'NONE', *, *, #7055, .F. ) ;
#5142=ORIENTED_EDGE ( 'NONE', *, *, #2923, .T. ) ;
#5144=AXIS2_PLACEMENT_3D ( 'NONE', #1036, #6995, #2548 ) ;
#5146=CARTESIAN_POINT ( 'NONE',  ( 0.000000000000000000, 38.99999999999993605, 0.000000000000000000 ) ) ;
#5147=VERTEX_POINT ( 'NONE', #3281 ) ;
#5151=CARTESIAN_POINT ( 'NONE',  ( -33.23540996127940872, 59.98874451312625666, -3.062309845534580077 ) ) ;
#5152=VECTOR ( 'NONE', #5627, 1000.000000000000000 ) ;
#5154=CYLINDRICAL_SURFACE ( 'NONE', #6222, 38.00000000000000711 ) ;
#5159=DIRECTION ( 'NONE',  ( 0.000000000000000000, 1.000000000000000000, 0.000000000000000000 ) ) ;
#5160=FACE_OUTER_BOUND ( 'NONE', #1943, .T. ) ;
#5165=VERTEX_POINT ( 'NONE', #291 ) ;
#5166=EDGE_CURVE ( 'NONE', #9301, #300, #9512, .T. ) ;
#5167=CARTESIAN_POINT ( 'NONE',  ( -2.304377683636469277E-13, 54.99999999999999289, 33.00000000000000711 ) ) ;
#5168=DIRECTION ( 'NONE',  ( 1.000000000000000000, 0.000000000000000000, 0.000000000000000000 ) ) ;
#5170=EDGE_CURVE ( 'NONE', #9011, #2376, #5842, .T. ) ;
#5172=EDGE_CURVE ( 'NONE', #4095, #4849, #384, .T. ) ;
#5173=CARTESIAN_POINT ( 'NONE',  ( 23.54759692749571087, 39.99999999999999289, -18.58791755254458167 ) ) ;
#5174=CARTESIAN_POINT ( 'NONE',  ( 0.000000000000000000, 59.99999999999999289, -30.00000000000000711 ) ) ;
#5178=CARTESIAN_POINT ( 'NONE',  ( 0.000000000000000000, 39.99999999999999289, 0.000000000000000000 ) ) ;
#5179=CARTESIAN_POINT ( 'NONE',  ( 31.18357922838634266, 54.99999999999999289, 10.79742499427304381 ) ) ;
#5182=CARTESIAN_POINT ( 'NONE',  ( 0.000000000000000000, 30.00000000000000000, 0.000000000000000000 ) ) ;
#5183=ORIENTED_EDGE ( 'NONE', *, *, #5947, .F. ) ;
#5187=DIRECTION ( 'NONE',  ( 0.000000000000000000, 0.000000000000000000, -1.000000000000000000 ) ) ;
#5194=VERTEX_POINT ( 'NONE', #3337 ) ;
#5195=LINE ( 'NONE', #4555, #887 ) ;
#5197=FACE_OUTER_BOUND ( 'NONE', #9541, .T. ) ;
#5198=ORIENTED_EDGE ( 'NONE', *, *, #8614, .F. ) ;
#5205=VERTEX_POINT ( 'NONE', #2638 ) ;
#5206=DIRECTION ( 'NONE',  ( 0.000000000000000000, 0.000000000000000000, -1.000000000000000000 ) ) ;
#5207=LINE ( 'NONE', #6480, #4486 ) ;
#5216=ADVANCED_FACE ( 'NONE', ( #8578 ), #1806, .T. ) ;
#5217=CARTESIAN_POINT ( 'NONE',  ( 0.000000000000000000, 54.99999999999999289, 0.000000000000000000 ) ) ;
#5220=AXIS2_PLACEMENT_3D ( 'NONE', #6587, #5116, #1362 ) ;
#5222=FACE_OUTER_BOUND ( 'NONE', #4280, .T. ) ;
#5226=EDGE_CURVE ( 'NONE', #2408, #742, #1594, .T. ) ;
#5230=VERTEX_POINT ( 'NONE', #7135 ) ;
#5231=DIRECTION ( 'NONE',  ( 0.5773502691896205130, 0.5773502691896365002, -0.5773502691896204020 ) ) ;
#5233=ORIENTED_EDGE ( 'NONE', *, *, #790, .F. ) ;
#5243=FACE_OUTER_BOUND ( 'NONE', #2804, .T. ) ;
#5245=ORIENTED_EDGE ( 'NONE', *, *, #4088, .T. ) ;
#5246=CARTESIAN_POINT ( 'NONE',  ( -33.06426808735054124, 49.99999999999999289, -5.562309845534581854 ) ) ;
#5252=AXIS2_PLACEMENT_3D ( 'NONE', #9234, #1763, #342 ) ;
#5254=CARTESIAN_POINT ( 'NONE',  ( -5.562309845551829390, 59.00253480853272947, 35.56426808735054834 ) ) ;
#5256=AXIS2_PLACEMENT_3D ( 'NONE', #1445, #1354, #4469 ) ;
#5258=ORIENTED_EDGE ( 'NONE', *, *, #8730, .T. ) ;
#5260=CARTESIAN_POINT ( 'NONE',  ( 30.00000000000000711, 59.99999999999999289, 1.047444401652940259E-13 ) ) ;
#5261=VECTOR ( 'NONE', #6533, 1000.000000000000000 ) ;
#5262=FACE_OUTER_BOUND ( 'NONE', #7050, .T. ) ;
#5263=CARTESIAN_POINT ( 'NONE',  ( 23.54759692749571443, 39.99999999999999289, -18.58791755254457811 ) ) ;
#5265=CARTESIAN_POINT ( 'NONE',  ( 0.000000000000000000, 39.99999999999999289, 0.000000000000000000 ) ) ;
#5267=DIRECTION ( 'NONE',  ( 0.000000000000000000, 1.000000000000000000, 0.000000000000000000 ) ) ;
#5269=FACE_OUTER_BOUND ( 'NONE', #8013, .T. ) ;
#5272=CARTESIAN_POINT ( 'NONE',  ( -4.000000000000005329, 30.00000000000000000, -29.00000000000000355 ) ) ;
#5274=VECTOR ( 'NONE', #7539, 1000.000000000000000 ) ;
#5276=DIRECTION ( 'NONE',  ( 0.000000000000000000, 1.000000000000000000, 0.000000000000000000 ) ) ;
#5280=ORIENTED_EDGE ( 'NONE', *, *, #9403, .T. ) ;
#5283=VECTOR ( 'NONE', #2787, 1000.000000000000114 ) ;
#5290=CIRCLE ( 'NONE', #2754, 2.500000000000002220 ) ;
#5293=ORIENTED_EDGE ( 'NONE', *, *, #5138, .T. ) ;
#5296=DIRECTION ( 'NONE',  ( -0.000000000000000000, -1.000000000000000000, -0.000000000000000000 ) ) ;
#5303=FACE_OUTER_BOUND ( 'NONE', #1493, .T. ) ;
#5304=AXIS2_PLACEMENT_3D ( 'NONE', #1098, #2566, #1881 ) ;
#5305=ADVANCED_FACE ( 'NONE', ( #2041 ), #5807, .F. ) ;
#5307=AXIS2_PLACEMENT_3D ( 'NONE', #9549, #6578, #5798 ) ;
#5309=CIRCLE ( 'NONE', #5918, 25.00000000000000000 ) ;
#5312=ORIENTED_EDGE ( 'NONE', *, *, #1533, .F. ) ;
#5313=ORIENTED_EDGE ( 'NONE', *, *, #9581, .F. ) ;
#5314=CARTESIAN_POINT ( 'NONE',  ( 0.000000000000000000, 54.99999999999999289, -33.00000000000000711 ) ) ;
#5316=CARTESIAN_POINT ( 'NONE',  ( 26.33333333333338544, 26.33333333333327886, 1.333333333333379001 ) ) ;
#5317=VECTOR ( 'NONE', #7948, 1000.000000000000000 ) ;
#5320=EDGE_LOOP ( 'NONE', ( #1634, #9295, #7744, #4775, #5680, #9338, #6745, #7797, #5428, #4370, #5139 ) ) ;
#5321=CARTESIAN_POINT ( 'NONE',  ( 0.000000000000000000, 30.00000000000000000, 0.000000000000000000 ) ) ;
#5324=DIRECTION ( 'NONE',  ( 0.000000000000000000, 0.000000000000000000, 1.000000000000000000 ) ) ;
#5340=ORIENTED_EDGE ( 'NONE', *, *, #3525, .T. ) ;
#5346=CARTESIAN_POINT ( 'NONE',  ( 25.51470164434615029, 30.00000000000000000, 5.000000000000000888 ) ) ;
#5347=ORIENTED_EDGE ( 'NONE', *, *, #5226, .F. ) ;
#5351=FACE_OUTER_BOUND ( 'NONE', #6804, .T. ) ;
#5353=CARTESIAN_POINT ( 'NONE',  ( -24.67792535850613334, 28.99999999999997158, 4.000000000000009770 ) ) ;
#5358=EDGE_CURVE ( 'NONE', #4065, #8074, #6938, .T. ) ;
#5361=PLANE ( 'NONE',  #1648 ) ;
#5365=CIRCLE ( 'NONE', #2347, 4.999999999999997335 ) ;
#5367=ORIENTED_EDGE ( 'NONE', *, *, #538, .F. ) ;
#5369=CARTESIAN_POINT ( 'NONE',  ( 0.000000000000000000, 39.99999999999999289, 0.000000000000000000 ) ) ;
#5370=CARTESIAN_POINT ( 'NONE',  ( -5.562309845551829390, 59.00253480853272947, 35.56426808735054834 ) ) ;
#5373=CARTESIAN_POINT ( 'NONE',  ( 8.063708916478045552, 59.93271281907998826, -32.87005020308307479 ) ) ;
#5374=DIRECTION ( 'NONE',  ( 0.000000000000000000, 0.000000000000000000, 1.000000000000000000 ) ) ;
#5377=ORIENTED_EDGE ( 'NONE', *, *, #8614, .T. ) ;
#5378=AXIS2_PLACEMENT_3D ( 'NONE', #6974, #1704, #4581 ) ;
#5379=CARTESIAN_POINT ( 'NONE',  ( 18.58791755254457811, 59.99999999999999289, 23.54759692749571443 ) ) ;
#5381=ORIENTED_EDGE ( 'NONE', *, *, #9033, .F. ) ;
#5384=DIRECTION ( 'NONE',  ( 0.7849198975831889191, -0.000000000000000000, -0.6195972517514874989 ) ) ;
#5393=EDGE_CURVE ( 'NONE', #2908, #1478, #1429, .T. ) ;
#5400=ORIENTED_EDGE ( 'NONE', *, *, #1606, .T. ) ;
#5401=CARTESIAN_POINT ( 'NONE',  ( -29.82695610816121956, 59.99999999999999289, 23.54469556655648432 ) ) ;
#5402=CARTESIAN_POINT ( 'NONE',  ( 24.96033808169876878, 29.33187429063046991, -4.331874290630493896 ) ) ;
#5405=ORIENTED_EDGE ( 'NONE', *, *, #9018, .F. ) ;
#5408=ORIENTED_EDGE ( 'NONE', *, *, #5936, .T. ) ;
#5409=ORIENTED_EDGE ( 'NONE', *, *, #5166, .T. ) ;
#5412=ADVANCED_FACE ( 'NONE', ( #2881 ), #6465, .T. ) ;
#5413=EDGE_CURVE ( 'NONE', #1128, #2408, #183, .T. ) ;
#5416=ADVANCED_FACE ( 'NONE', ( #768 ), #5361, .F. ) ;
#5417=PLANE ( 'NONE',  #8081 ) ;
#5421=DIRECTION ( 'NONE',  ( 0.000000000000000000, 0.000000000000000000, 1.000000000000000000 ) ) ;
#5422=VECTOR ( 'NONE', #3043, 1000.000000000000000 ) ;
#5425=DIRECTION ( 'NONE',  ( 0.000000000000000000, 0.000000000000000000, 1.000000000000000000 ) ) ;
#5426=LINE ( 'NONE', #7078, #2381 ) ;
#5428=ORIENTED_EDGE ( 'NONE', *, *, #2796, .F. ) ;
#5431=ORIENTED_EDGE ( 'NONE', *, *, #9215, .F. ) ;
#5435=VECTOR ( 'NONE', #9270, 1000.000000000000000 ) ;
#5439=LINE ( 'NONE', #8448, #5134 ) ;
#5440=ORIENTED_EDGE ( 'NONE', *, *, #3530, .F. ) ;
#5443=CARTESIAN_POINT ( 'NONE',  ( -28.34870838944214100, 39.99999999999999289, -9.815840903884556212 ) ) ;
#5444=VECTOR ( 'NONE', #7247, 1000.000000000000000 ) ;
#5445=DIRECTION ( 'NONE',  ( 0.9444444444444443088, -0.000000000000000000, -0.3286710990610907657 ) ) ;
#5448=LINE ( 'NONE', #6954, #900 ) ;
#5453=AXIS2_PLACEMENT_3D ( 'NONE', #6215, #9249, #1330 ) ;
#5456=FACE_OUTER_BOUND ( 'NONE', #841, .T. ) ;
#5464=FACE_OUTER_BOUND ( 'NONE', #2111, .T. ) ;
#5466=CARTESIAN_POINT ( 'NONE',  ( 18.58791755254457811, 39.99999999999999289, 23.54759692749571443 ) ) ;
#5467=VECTOR ( 'NONE', #6834, 999.9999999999998863 ) ;
#5469=CARTESIAN_POINT ( 'NONE',  ( 0.000000000000000000, -50.91168824543140659, 0.000000000000000000 ) ) ;
#5474=CARTESIAN_POINT ( 'NONE',  ( 3.106744199778904925, 59.95265069314689299, -33.56539760714087350 ) ) ;
#5475=CIRCLE ( 'NONE', #9104, 25.00000000000000000 ) ;
#5476=FACE_OUTER_BOUND ( 'NONE', #494, .T. ) ;
#5477=FACE_OUTER_BOUND ( 'NONE', #8377, .T. ) ;
#5478=EDGE_CURVE ( 'NONE', #8947, #5781, #9066, .T. ) ;
#5481=LINE ( 'NONE', #8387, #7806 ) ;
#5488=CARTESIAN_POINT ( 'NONE',  ( 28.34870838944214100, 59.99999999999999289, 9.815840903884559765 ) ) ;
#5489=ORIENTED_EDGE ( 'NONE', *, *, #5619, .T. ) ;
#5493=ORIENTED_EDGE ( 'NONE', *, *, #4154, .T. ) ;
#5496=ORIENTED_EDGE ( 'NONE', *, *, #3441, .T. ) ;
#5499=B_SPLINE_CURVE_WITH_KNOTS ( 'NONE', 3,
 ( #2146, #8084, #1226, #3487, #9518, #2002 ),
 .UNSPECIFIED., .F., .F.,
 ( 4, 2, 4 ),
 ( 0.000000000000000000, 0.0005212762617847652939, 0.001042552523569530588 ),
 .UNSPECIFIED. ) ;
#5500=ORIENTED_EDGE ( 'NONE', *, *, #5358, .F. ) ;
#5501=DIRECTION ( 'NONE',  ( 1.000000000000000000, 0.000000000000000000, -1.084202172485503448E-16 ) ) ;
#5505=CARTESIAN_POINT ( 'NONE',  ( -34.30759795839968262, 59.50675430643739361, -7.737048950318285101 ) ) ;
#5507=DIRECTION ( 'NONE',  ( 0.000000000000000000, -1.000000000000000000, 0.000000000000000000 ) ) ;
#5508=ORIENTED_EDGE ( 'NONE', *, *, #8130, .F. ) ;
#5514=ADVANCED_FACE ( 'NONE', ( #5351 ), #3815, .F. ) ;
#5516=CARTESIAN_POINT ( 'NONE',  ( 3.850561375233632511, 59.53730689706333834, -34.89414954626303000 ) ) ;
#5517=FACE_OUTER_BOUND ( 'NONE', #5022, .T. ) ;
#5521=VECTOR ( 'NONE', #4423, 1000.000000000000114 ) ;
#5523=CIRCLE ( 'NONE', #8196, 39.00000000000002132 ) ;
#5524=LINE ( 'NONE', #4879, #862 ) ;
#5529=EDGE_CURVE ( 'NONE', #2376, #2208, #6866, .T. ) ;
#5531=ADVANCED_FACE ( 'NONE', ( #5303 ), #9695, .T. ) ;
#5533=EDGE_CURVE ( 'NONE', #8554, #3288, #3113, .T. ) ;
#5536=CARTESIAN_POINT ( 'NONE',  ( -12.43339847825378719, 54.99999999999999289, 35.90836395996003461 ) ) ;
#5538=ORIENTED_EDGE ( 'NONE', *, *, #9095, .F. ) ;
#5539=DIRECTION ( 'NONE',  ( 0.000000000000000000, 0.000000000000000000, 1.000000000000000000 ) ) ;
#5541=CARTESIAN_POINT ( 'NONE',  ( 35.88888888888889284, 54.99999999999999289, -12.48950176432140502 ) ) ;
#5543=DIRECTION ( 'NONE',  ( -1.000000000000000000, 0.000000000000000000, 0.000000000000000000 ) ) ;
#5544=DIRECTION ( 'NONE',  ( -0.7849198975831893632, -0.000000000000000000, 0.6195972517514870548 ) ) ;
#5549=EDGE_LOOP ( 'NONE', ( #2304, #4868, #593, #9699 ) ) ;
#5550=DIRECTION ( 'NONE',  ( 0.000000000000000000, 1.000000000000000000, 0.000000000000000000 ) ) ;
#5551=ORIENTED_EDGE ( 'NONE', *, *, #2180, .F. ) ;
#5557=DIRECTION ( 'NONE',  ( -0.000000000000000000, -1.000000000000000000, -0.000000000000000000 ) ) ;
#5559=DIRECTION ( 'NONE',  ( 0.000000000000000000, 1.000000000000000000, 0.000000000000000000 ) ) ;
#5568=LINE ( 'NONE', #9367, #3623 ) ;
#5571=ORIENTED_EDGE ( 'NONE', *, *, #8234, .T. ) ;
#5573=CARTESIAN_POINT ( 'NONE',  ( -5.000000000000006217, 30.00000000000000000, -25.51470164434615029 ) ) ;
#5576=CARTESIAN_POINT ( 'NONE',  ( 8.673617379884035472E-16, 30.00000000000000000, 4.000000000000004441 ) ) ;
#5577=DIRECTION ( 'NONE',  ( 0.000000000000000000, 0.000000000000000000, 1.000000000000000000 ) ) ;
#5581=EDGE_CURVE ( 'NONE', #3464, #427, #9327, .T. ) ;
#5585=EDGE_CURVE ( 'NONE', #5689, #9409, #6757, .T. ) ;
#5586=ORIENTED_EDGE ( 'NONE', *, *, #6720, .F. ) ;
#5587=AXIS2_PLACEMENT_3D ( 'NONE', #8982, #5276, #2151 ) ;
#5588=CARTESIAN_POINT ( 'NONE',  ( -4.999999999999999112, 30.00000000000000000, 30.00000000000000711 ) ) ;
#5590=VECTOR ( 'NONE', #9055, 1000.000000000000114 ) ;
#5594=ADVANCED_FACE ( 'NONE', ( #8643 ), #3860, .T. ) ;
#5596=FACE_OUTER_BOUND ( 'NONE', #9532, .T. ) ;
#5597=ORIENTED_EDGE ( 'NONE', *, *, #4438, .F. ) ;
#5598=VERTEX_POINT ( 'NONE', #6500 ) ;
#5599=ADVANCED_FACE ( 'NONE', ( #1279 ), #2750, .T. ) ;
#5601=VECTOR ( 'NONE', #6953, 1000.000000000000114 ) ;
#5602=DIRECTION ( 'NONE',  ( 0.000000000000000000, 0.000000000000000000, 1.000000000000000000 ) ) ;
#5605=AXIS2_PLACEMENT_3D ( 'NONE', #2357, #9098, #1631 ) ;
#5606=CIRCLE ( 'NONE', #8132, 26.00000000000000355 ) ;
#5609=AXIS2_PLACEMENT_3D ( 'NONE', #3084, #3740, #5324 ) ;
#5611=ORIENTED_EDGE ( 'NONE', *, *, #6224, .T. ) ;
#5616=FACE_OUTER_BOUND ( 'NONE', #4907, .T. ) ;
#5618=AXIS2_PLACEMENT_3D ( 'NONE', #1687, #1042, #3202 ) ;
#5619=EDGE_CURVE ( 'NONE', #8688, #3761, #8746, .T. ) ;
#5620=AXIS2_PLACEMENT_3D ( 'NONE', #5246, #1735, #6168 ) ;
#5621=ORIENTED_EDGE ( 'NONE', *, *, #1421, .F. ) ;
#5622=FACE_OUTER_BOUND ( 'NONE', #1578, .T. ) ;
#5625=ORIENTED_EDGE ( 'NONE', *, *, #1544, .T. ) ;
#5626=DIRECTION ( 'NONE',  ( 0.000000000000000000, 0.000000000000000000, 1.000000000000000000 ) ) ;
#5627=DIRECTION ( 'NONE',  ( -0.000000000000000000, -1.000000000000000000, -0.000000000000000000 ) ) ;
#5629=DIRECTION ( 'NONE',  ( -0.000000000000000000, 1.000000000000000000, -0.000000000000000000 ) ) ;
#5637=LINE ( 'NONE', #8649, #2271 ) ;
#5639=CARTESIAN_POINT ( 'NONE',  ( 32.05305536707737701, 59.99999999999999289, 7.848671329280705322 ) ) ;
#5642=CARTESIAN_POINT ( 'NONE',  ( 20.99999999999999645, 0.000000000000000000, -4.000000000000006217 ) ) ;
#5647=ORIENTED_EDGE ( 'NONE', *, *, #3352, .T. ) ;
#5649=ORIENTED_EDGE ( 'NONE', *, *, #5948, .T. ) ;
#5651=CARTESIAN_POINT ( 'NONE',  ( 33.06426808735053413, 59.89212256466219486, 8.062309845534588959 ) ) ;
#5654=EDGE_CURVE ( 'NONE', #504, #6089, #7902, .T. ) ;
#5655=FACE_OUTER_BOUND ( 'NONE', #815, .T. ) ;
#5656=EDGE_CURVE ( 'NONE', #1193, #3167, #4247, .T. ) ;
#5662=CYLINDRICAL_SURFACE ( 'NONE', #270, 2.500000000000002220 ) ;
#5665=CARTESIAN_POINT ( 'NONE',  ( 23.54759692749571443, 59.99999999999999289, -18.58791755254457811 ) ) ;
#5669=LINE ( 'NONE', #339, #3155 ) ;
#5674=CARTESIAN_POINT ( 'NONE',  ( -28.33333333333344939, 59.99999999999999289, 9.860132971832396009 ) ) ;
#5676=CARTESIAN_POINT ( 'NONE',  ( 0.000000000000000000, 28.99999999999997158, -29.00000000000000355 ) ) ;
#5677=AXIS2_PLACEMENT_3D ( 'NONE', #7687, #3421, #5421 ) ;
#5679=FACE_OUTER_BOUND ( 'NONE', #604, .T. ) ;
#5680=ORIENTED_EDGE ( 'NONE', *, *, #8991, .F. ) ;
#5684=VECTOR ( 'NONE', #6289, 1000.000000000000000 ) ;
#5685=CARTESIAN_POINT ( 'NONE',  ( 0.000000000000000000, 28.99999999999997158, 29.00000000000000355 ) ) ;
#5686=CARTESIAN_POINT ( 'NONE',  ( -23.54469556655647722, 54.99999999999999289, -29.82695610816121956 ) ) ;
#5688=AXIS2_PLACEMENT_3D ( 'NONE', #5944, #8966, #1700 ) ;
#5689=VERTEX_POINT ( 'NONE', #8041 ) ;
#5695=EDGE_CURVE ( 'NONE', #5165, #8947, #2647, .T. ) ;
#5697=DIRECTION ( 'NONE',  ( 0.000000000000000000, 0.000000000000000000, -1.000000000000000000 ) ) ;
#5700=DIRECTION ( 'NONE',  ( -1.000000000000000000, 0.000000000000000000, 0.000000000000000000 ) ) ;
#5701=CARTESIAN_POINT ( 'NONE',  ( -3.060768115627992003, 59.99034304420147379, 33.21665709534246957 ) ) ;
#5712=AXIS2_PLACEMENT_3D ( 'NONE', #7574, #73, #3162 ) ;
#5714=DIRECTION ( 'NONE',  ( 0.9449569463147374782, 0.000000000000000000, 0.3271946967961527619 ) ) ;
#5715=FACE_OUTER_BOUND ( 'NONE', #8207, .T. ) ;
#5716=ORIENTED_EDGE ( 'NONE', *, *, #1533, .T. ) ;
#5724=DIRECTION ( 'NONE',  ( 0.000000000000000000, 0.000000000000000000, 1.000000000000000000 ) ) ;
#5725=VECTOR ( 'NONE', #8836, 1000.000000000000000 ) ;
#5737=CARTESIAN_POINT ( 'NONE',  ( 0.000000000000000000, -50.91168824543140659, 17.99999999999999645 ) ) ;
#5738=EDGE_LOOP ( 'NONE', ( #3049, #1250, #6906, #863 ) ) ;
#5740=ORIENTED_EDGE ( 'NONE', *, *, #9263, .T. ) ;
#5743=CARTESIAN_POINT ( 'NONE',  ( -33.06426808735054124, 49.99999999999999289, -3.062309845534580077 ) ) ;
#5746=AXIS2_PLACEMENT_3D ( 'NONE', #7742, #6939, #9232 ) ;
#5747=ORIENTED_EDGE ( 'NONE', *, *, #2851, .T. ) ;
#5748=DIRECTION ( 'NONE',  ( 0.000000000000000000, 0.000000000000000000, 1.000000000000000000 ) ) ;
#5751=DIRECTION ( 'NONE',  ( -0.000000000000000000, -1.000000000000000000, -0.000000000000000000 ) ) ;
#5756=CYLINDRICAL_SURFACE ( 'NONE', #4746, 2.499999999999998668 ) ;
#5773=AXIS2_PLACEMENT_3D ( 'NONE', #92, #4536, #9715 ) ;
#5775=EDGE_CURVE ( 'NONE', #2914, #9233, #3037, .T. ) ;
#5776=EDGE_CURVE ( 'NONE', #4788, #71, #1021, .T. ) ;
#5777=CIRCLE ( 'NONE', #2772, 19.00000000000005684 ) ;
#5780=PLANE ( 'NONE',  #1185 ) ;
#5781=VERTEX_POINT ( 'NONE', #2053 ) ;
#5785=AXIS2_PLACEMENT_3D ( 'NONE', #1091, #6318, #4756 ) ;
#5786=DIRECTION ( 'NONE',  ( -0.000000000000000000, -1.000000000000000000, -0.000000000000000000 ) ) ;
#5791=CARTESIAN_POINT ( 'NONE',  ( -33.72911585420148128, 59.92558239856793278, -3.146586008005425761 ) ) ;
#5793=DIRECTION ( 'NONE',  ( 0.000000000000000000, 0.000000000000000000, -1.000000000000000000 ) ) ;
#5795=ORIENTED_EDGE ( 'NONE', *, *, #2672, .T. ) ;
#5798=DIRECTION ( 'NONE',  ( 0.000000000000000000, 0.000000000000000000, 1.000000000000000000 ) ) ;
#5800=ORIENTED_EDGE ( 'NONE', *, *, #8959, .T. ) ;
#5803=ORIENTED_EDGE ( 'NONE', *, *, #5695, .T. ) ;
#5807=PLANE ( 'NONE',  #7584 ) ;
#5810=CARTESIAN_POINT ( 'NONE',  ( -5.000000000000006217, 30.00000000000000000, -25.51470164434615029 ) ) ;
#5811=ORIENTED_EDGE ( 'NONE', *, *, #74, .F. ) ;
#5812=CARTESIAN_POINT ( 'NONE',  ( 0.000000000000000000, 30.00000000000000000, 0.000000000000000000 ) ) ;
#5819=LINE ( 'NONE', #2845, #4811 ) ;
#5825=EDGE_CURVE ( 'NONE', #167, #2908, #3941, .T. ) ;
#5829=AXIS2_PLACEMENT_3D ( 'NONE', #8576, #1855, #7692 ) ;
#5832=EDGE_LOOP ( 'NONE', ( #2121, #6617, #7921, #8441 ) ) ;
#5833=DIRECTION ( 'NONE',  ( -1.533293416683393860E-16, 0.7071067811865376918, -0.7071067811865573427 ) ) ;
#5835=CARTESIAN_POINT ( 'NONE',  ( 9.815840903884561541, 39.99999999999999289, -28.34870838944214100 ) ) ;
#5839=CARTESIAN_POINT ( 'NONE',  ( 0.000000000000000000, 54.99999999999999289, 0.000000000000000000 ) ) ;
#5842=CIRCLE ( 'NONE', #6307, 38.00000000000000711 ) ;
#5843=ORIENTED_EDGE ( 'NONE', *, *, #8735, .F. ) ;
#5845=VERTEX_POINT ( 'NONE', #196 ) ;
#5847=DIRECTION ( 'NONE',  ( 0.000000000000000000, 0.000000000000000000, -1.000000000000000000 ) ) ;
#5849=( LENGTH_UNIT ( ) NAMED_UNIT ( * ) SI_UNIT ( .MILLI., .METRE. ) );
#5851=CARTESIAN_POINT ( 'NONE',  ( -33.06426808735054124, 49.99999999999999289, -8.062309845534583630 ) ) ;
#5855=VERTEX_POINT ( 'NONE', #8434 ) ;
#5862=FACE_OUTER_BOUND ( 'NONE', #1384, .T. ) ;
#5863=VERTEX_POINT ( 'NONE', #3283 ) ;
#5867=ORIENTED_EDGE ( 'NONE', *, *, #1088, .F. ) ;
#5868=CARTESIAN_POINT ( 'NONE',  ( 24.67792535850613334, 30.00000000000000000, -4.000000000000006217 ) ) ;
#5880=ORIENTED_EDGE ( 'NONE', *, *, #4987, .F. ) ;
#5884=DIRECTION ( 'NONE',  ( 0.000000000000000000, 0.000000000000000000, 1.000000000000000000 ) ) ;
#5887=ORIENTED_EDGE ( 'NONE', *, *, #1124, .T. ) ;
#5892=CARTESIAN_POINT ( 'NONE',  ( -5.000000000000006217, 30.00000000000000000, -30.00000000000000711 ) ) ;
#5894=CARTESIAN_POINT ( 'NONE',  ( 0.000000000000000000, 59.99999999999999289, -30.00000000000000711 ) ) ;
#5896=CIRCLE ( 'NONE', #3693, 5.000000000000001776 ) ;
#5897=DIRECTION ( 'NONE',  ( -0.7849198975831889191, -0.000000000000000000, 0.6195972517514874989 ) ) ;
#5898=VERTEX_POINT ( 'NONE', #6105 ) ;
#5901=LINE ( 'NONE', #7394, #8001 ) ;
#5902=CARTESIAN_POINT ( 'NONE',  ( 20.99999999999999645, 28.99999999999997158, -4.000000000000006217 ) ) ;
#5904=CARTESIAN_POINT ( 'NONE',  ( 10.84614626901583634, 59.99999999999999289, 31.16666666666671759 ) ) ;
#5906=EDGE_CURVE ( 'NONE', #3718, #4111, #2106, .T. ) ;
#5912=AXIS2_PLACEMENT_3D ( 'NONE', #5265, #2291, #2093 ) ;
#5914=DIRECTION ( 'NONE',  ( 2.168404344971006649E-16, 0.000000000000000000, 1.000000000000000000 ) ) ;
#5916=ORIENTED_EDGE ( 'NONE', *, *, #8248, .F. ) ;
#5917=LINE ( 'NONE', #4359, #2391 ) ;
#5918=AXIS2_PLACEMENT_3D ( 'NONE', #96, #3085, #5425 ) ;
#5926=CARTESIAN_POINT ( 'NONE',  ( -34.95336322954870667, 59.50565096299369827, -3.917041198934857693 ) ) ;
#5927=TOROIDAL_SURFACE ( 'NONE', #2301, 33.00000000000000711, 5.000000000000000000 ) ;
#5929=CARTESIAN_POINT ( 'NONE',  ( 34.60286690457041914, 59.67177527313210561, 3.585274540811282051 ) ) ;
#5930=ORIENTED_EDGE ( 'NONE', *, *, #983, .T. ) ;
#5936=EDGE_CURVE ( 'NONE', #9170, #3887, #5481, .T. ) ;
#5944=CARTESIAN_POINT ( 'NONE',  ( 0.000000000000000000, 39.99999999999999289, 0.000000000000000000 ) ) ;
#5945=EDGE_CURVE ( 'NONE', #3216, #9301, #7740, .T. ) ;
#5946=CARTESIAN_POINT ( 'NONE',  ( 25.90235662024523577, 54.99999999999999289, -20.44670930779909312 ) ) ;
#5947=EDGE_CURVE ( 'NONE', #1652, #9574, #6059, .T. ) ;
#5948=EDGE_CURVE ( 'NONE', #8562, #5205, #405, .T. ) ;
#5949=FACE_OUTER_BOUND ( 'NONE', #7062, .T. ) ;
#5953=CYLINDRICAL_SURFACE ( 'NONE', #3174, 17.99999999999999645 ) ;
#5958=DIRECTION ( 'NONE',  ( 1.000000000000000000, 0.000000000000000000, -1.084202172485503448E-16 ) ) ;
#5963=ORIENTED_EDGE ( 'NONE', *, *, #7218, .F. ) ;
#5967=CARTESIAN_POINT ( 'NONE',  ( -33.06426808735054124, 49.99999999999999289, -8.062309845534585406 ) ) ;
#5970=DIRECTION ( 'NONE',  ( 0.000000000000000000, 0.000000000000000000, 1.000000000000000000 ) ) ;
#5971=ORIENTED_EDGE ( 'NONE', *, *, #106, .F. ) ;
#5979=CARTESIAN_POINT ( 'NONE',  ( -9.815840903884557989, 59.99999999999999289, 28.34870838944214455 ) ) ;
#5982=ORIENTED_EDGE ( 'NONE', *, *, #4213, .T. ) ;
#5989=CARTESIAN_POINT ( 'NONE',  ( -4.665243217607704551, 29.66524321760768501, -25.23917843705063646 ) ) ;
#5993=PLANE ( 'NONE',  #28 ) ;
#6003=CARTESIAN_POINT ( 'NONE',  ( 0.000000000000000000, 30.99999999999998579, -40.00000000000000711 ) ) ;
#6007=VECTOR ( 'NONE', #330, 1000.000000000000114 ) ;
#6014=VERTEX_POINT ( 'NONE', #6345 ) ;
#6016=CYLINDRICAL_SURFACE ( 'NONE', #1415, 30.00000000000001066 ) ;
#6018=ORIENTED_EDGE ( 'NONE', *, *, #1897, .F. ) ;
#6024=ADVANCED_FACE ( 'NONE', ( #8727 ), #9365, .T. ) ;
#6025=CARTESIAN_POINT ( 'NONE',  ( 0.000000000000000000, 0.000000000000000000, 0.000000000000000000 ) ) ;
#6027=CARTESIAN_POINT ( 'NONE',  ( -7.123219286842091158, 59.18149658568252391, 35.02766888370170051 ) ) ;
#6028=ORIENTED_EDGE ( 'NONE', *, *, #1694, .F. ) ;
#6030=PRODUCT_DEFINITION_CONTEXT ( 'detailed design', #1394, 'design' ) ;
#6040=DIRECTION ( 'NONE',  ( 2.168404344971006649E-16, -0.000000000000000000, 1.000000000000000000 ) ) ;
#6047=EDGE_CURVE ( 'NONE', #9236, #156, #6491, .T. ) ;
#6049=CIRCLE ( 'NONE', #871, 30.00000000000000711 ) ;
#6050=EDGE_CURVE ( 'NONE', #982, #1104, #7936, .T. ) ;
#6051=DIRECTION ( 'NONE',  ( 7.666467083416970531E-17, 0.7071067811865375807, 0.7071067811865574537 ) ) ;
#6052=CARTESIAN_POINT ( 'NONE',  ( -3.999999999999999112, 0.000000000000000000, 24.67792535850613334 ) ) ;
#6053=PRODUCT ( 'Metal Body for Mounting Threaded Chasers', 'Metal Body for Mounting Threaded Chasers', '', ( #63 ) ) ;
#6058=VECTOR ( 'NONE', #8899, 1000.000000000000000 ) ;
#6059=CIRCLE ( 'NONE', #9074, 5.000000000000000000 ) ;
#6062=CARTESIAN_POINT ( 'NONE',  ( 0.000000000000000000, 59.99999999999999289, 0.000000000000000000 ) ) ;
#6070=AXIS2_PLACEMENT_3D ( 'NONE', #9406, #1100, #3426 ) ;
#6072=ORIENTED_EDGE ( 'NONE', *, *, #4496, .F. ) ;
#6076=ORIENTED_EDGE ( 'NONE', *, *, #2991, .F. ) ;
#6077=CARTESIAN_POINT ( 'NONE',  ( 4.000000000000007994, 0.000000000000000000, 24.67792535850613334 ) ) ;
#6080=DIRECTION ( 'NONE',  ( -0.000000000000000000, 1.000000000000000000, -0.000000000000000000 ) ) ;
#6082=DIRECTION ( 'NONE',  ( -0.000000000000000000, -1.000000000000000000, -0.000000000000000000 ) ) ;
#6085=ADVANCED_BREP_SHAPE_REPRESENTATION ( '', ( #6272, #6314 ), #2843 ) ;
#6087=CARTESIAN_POINT ( 'NONE',  ( -8.063708916478040223, 59.93271281907998826, 32.87005020308307479 ) ) ;
#6089=VERTEX_POINT ( 'NONE', #1906 ) ;
#6094=CIRCLE ( 'NONE', #9569, 5.000000000000001776 ) ;
#6095=DIRECTION ( 'NONE',  ( 0.000000000000000000, 0.000000000000000000, 1.000000000000000000 ) ) ;
#6097=DIRECTION ( 'NONE',  ( -0.9449569463147374782, 0.000000000000000000, -0.3271946967961527619 ) ) ;
#6098=FACE_OUTER_BOUND ( 'NONE', #472, .T. ) ;
#6101=CARTESIAN_POINT ( 'NONE',  ( 4.397412886516829822, 59.29888504437717955, -35.28275170782140435 ) ) ;
#6105=CARTESIAN_POINT ( 'NONE',  ( -32.05305536707737701, 59.99999999999999289, -7.848671329280701769 ) ) ;
#6108=ORIENTED_EDGE ( 'NONE', *, *, #8735, .T. ) ;
#6111=ORIENTED_EDGE ( 'NONE', *, *, #4973, .F. ) ;
#6117=ORIENTED_EDGE ( 'NONE', *, *, #1841, .T. ) ;
#6127=DIRECTION ( 'NONE',  ( 0.000000000000000000, 1.000000000000000000, 0.000000000000000000 ) ) ;
#6130=ORIENTED_EDGE ( 'NONE', *, *, #2372, .T. ) ;
#6131=CARTESIAN_POINT ( 'NONE',  ( -7.989536001449261349, 59.73029374780620060, 33.69619452719667407 ) ) ;
#6133=CIRCLE ( 'NONE', #1875, 25.00000000000000000 ) ;
#6136=DIRECTION ( 'NONE',  ( -0.000000000000000000, 1.000000000000000000, -0.000000000000000000 ) ) ;
#6138=CIRCLE ( 'NONE', #1886, 4.999999999999997335 ) ;
#6139=EDGE_LOOP ( 'NONE', ( #6846, #8357 ) ) ;
#6144=CARTESIAN_POINT ( 'NONE',  ( 3.147661243663450126, 59.92470504718686897, -33.73534932023821398 ) ) ;
#6145=CARTESIAN_POINT ( 'NONE',  ( 4.653657836759942730E-15, 54.99999999999999289, -38.00000000000000711 ) ) ;
#6147=CARTESIAN_POINT ( 'NONE',  ( 0.000000000000000000, 59.99999999999999289, 0.000000000000000000 ) ) ;
#6149=VERTEX_POINT ( 'NONE', #334 ) ;
#6152=EDGE_CURVE ( 'NONE', #6918, #5598, #3338, .T. ) ;
#6153=AXIS2_PLACEMENT_3D ( 'NONE', #8684, #4094, #1908 ) ;
#6160=DIRECTION ( 'NONE',  ( 0.000000000000000000, 0.000000000000000000, 1.000000000000000000 ) ) ;
#6166=DIRECTION ( 'NONE',  ( -0.000000000000000000, 1.000000000000000000, -0.000000000000000000 ) ) ;
#6167=ORIENTED_EDGE ( 'NONE', *, *, #9384, .T. ) ;
#6168=DIRECTION ( 'NONE',  ( 0.000000000000000000, -0.000000000000000000, 1.000000000000000000 ) ) ;
#6171=CARTESIAN_POINT ( 'NONE',  ( 25.23917843705063646, 29.66524321760768501, -4.665243217607707216 ) ) ;
#6173=EDGE_CURVE ( 'NONE', #8145, #1128, #8129, .T. ) ;
#6178=CARTESIAN_POINT ( 'NONE',  ( -10.79742499427308289, 54.99999999999999289, 31.18357922838633201 ) ) ;
#6179=ORIENTED_EDGE ( 'NONE', *, *, #7007, .T. ) ;
#6181=ORIENTED_EDGE ( 'NONE', *, *, #5013, .F. ) ;
#6184=DIRECTION ( 'NONE',  ( -0.9449569463147374782, 0.000000000000000000, -0.3271946967961527619 ) ) ;
#6185=CARTESIAN_POINT ( 'NONE',  ( 0.000000000000000000, 30.00000000000000000, 0.000000000000000000 ) ) ;
#6186=EDGE_CURVE ( 'NONE', #1776, #2818, #8920, .T. ) ;
#6191=CYLINDRICAL_SURFACE ( 'NONE', #4887, 40.00000000000000711 ) ;
#6195=CARTESIAN_POINT ( 'NONE',  ( 5.562309845551833831, 59.00253480853272947, -35.56426808735054834 ) ) ;
#6198=DIRECTION ( 'NONE',  ( 0.000000000000000000, 0.000000000000000000, 1.000000000000000000 ) ) ;
#6204=LINE ( 'NONE', #7856, #4055 ) ;
#6205=EDGE_CURVE ( 'NONE', #7344, #9409, #8918, .T. ) ;
#6207=DIRECTION ( 'NONE',  ( -0.000000000000000000, -1.000000000000000000, -0.000000000000000000 ) ) ;
#6212=DIRECTION ( 'NONE',  ( 1.000000000000000000, 0.000000000000000000, -2.168404344971006649E-16 ) ) ;
#6214=VECTOR ( 'NONE', #8539, 1000.000000000000000 ) ;
#6215=CARTESIAN_POINT ( 'NONE',  ( 0.000000000000000000, 59.99999999999999289, 0.000000000000000000 ) ) ;
#6217=DIRECTION ( 'NONE',  ( 0.000000000000000000, 0.000000000000000000, 1.000000000000000000 ) ) ;
#6218=VERTEX_POINT ( 'NONE', #7338 ) ;
#6219=PRODUCT_DEFINITION_SHAPE ( 'NONE', 'NONE',  #1863 ) ;
#6220=DIRECTION ( 'NONE',  ( 0.000000000000000000, 1.000000000000000000, 0.000000000000000000 ) ) ;
#6222=AXIS2_PLACEMENT_3D ( 'NONE', #1391, #2774, #5793 ) ;
#6224=EDGE_CURVE ( 'NONE', #6218, #300, #3585, .T. ) ;
#6225=ORIENTED_EDGE ( 'NONE', *, *, #9297, .F. ) ;
#6226=CARTESIAN_POINT ( 'NONE',  ( 29.00000000000000355, 30.00000000000000000, 4.000000000000000000 ) ) ;
#6228=ORIENTED_EDGE ( 'NONE', *, *, #8364, .F. ) ;
#6233=EDGE_LOOP ( 'NONE', ( #123, #1541, #3820, #4227 ) ) ;
#6239=PLANE ( 'NONE',  #9039 ) ;
#6240=VECTOR ( 'NONE', #2817, 1000.000000000000000 ) ;
#6242=CARTESIAN_POINT ( 'NONE',  ( 18.58791755254457811, 59.99999999999999289, 23.54759692749571443 ) ) ;
#6245=CARTESIAN_POINT ( 'NONE',  ( -4.999999999999813483, 19.99999999999990408, -20.00000000000019185 ) ) ;
#6248=CARTESIAN_POINT ( 'NONE',  ( 0.000000000000000000, 59.99999999999999289, 0.000000000000000000 ) ) ;
#6249=EDGE_CURVE ( 'NONE', #8321, #9687, #9540, .T. ) ;
#6253=VECTOR ( 'NONE', #5714, 1000.000000000000114 ) ;
#6254=DIRECTION ( 'NONE',  ( 0.000000000000000000, -1.000000000000000000, 0.000000000000000000 ) ) ;
#6255=ORIENTED_EDGE ( 'NONE', *, *, #3414, .F. ) ;
#6257=DIRECTION ( 'NONE',  ( 0.000000000000000000, 0.000000000000000000, 1.000000000000000000 ) ) ;
#6258=ORIENTED_EDGE ( 'NONE', *, *, #6843, .T. ) ;
#6259=PLANE ( 'NONE',  #7454 ) ;
#6261=EDGE_CURVE ( 'NONE', #1692, #7344, #6630, .T. ) ;
#6266=CARTESIAN_POINT ( 'NONE',  ( -35.88888888888889284, 54.99999999999999289, 12.48950176432140857 ) ) ;
#6272=MANIFOLD_SOLID_BREP ( 'Chamfer4', #120 ) ;
#6273=ORIENTED_EDGE ( 'NONE', *, *, #5945, .T. ) ;
#6276=LINE ( 'NONE', #7169, #6388 ) ;
#6281=DIRECTION ( 'NONE',  ( -0.000000000000000000, 1.000000000000000000, -0.000000000000000000 ) ) ;
#6286=DIRECTION ( 'NONE',  ( -0.000000000000000000, -1.000000000000000000, -0.000000000000000000 ) ) ;
#6288=CARTESIAN_POINT ( 'NONE',  ( 0.000000000000000000, 39.99999999999999289, 0.000000000000000000 ) ) ;
#6289=DIRECTION ( 'NONE',  ( -1.000000000000000000, 0.000000000000000000, 0.000000000000000000 ) ) ;
#6292=EDGE_CURVE ( 'NONE', #9059, #8698, #8221, .T. ) ;
#6298=AXIS2_PLACEMENT_3D ( 'NONE', #5217, #624, #3783 ) ;
#6304=ORIENTED_EDGE ( 'NONE', *, *, #9461, .F. ) ;
#6307=AXIS2_PLACEMENT_3D ( 'NONE', #3439, #1948, #2736 ) ;
#6309=EDGE_CURVE ( 'NONE', #1104, #9236, #2282, .T. ) ;
#6310=FACE_OUTER_BOUND ( 'NONE', #6829, .T. ) ;
#6312=EDGE_LOOP ( 'NONE', ( #1893, #3368, #836, #3170, #4410 ) ) ;
#6313=CARTESIAN_POINT ( 'NONE',  ( 0.000000000000000000, 59.99999999999999289, 0.000000000000000000 ) ) ;
#6314=AXIS2_PLACEMENT_3D ( 'NONE', #9654, #2830, #5168 ) ;
#6315=ORIENTED_EDGE ( 'NONE', *, *, #988, .F. ) ;
#6318=DIRECTION ( 'NONE',  ( -0.000000000000000000, 1.000000000000000000, -0.000000000000000000 ) ) ;
#6322=VECTOR ( 'NONE', #4684, 1000.000000000000000 ) ;
#6326=ORIENTED_EDGE ( 'NONE', *, *, #3270, .F. ) ;
#6331=B_SPLINE_CURVE_WITH_KNOTS ( 'NONE', 3,
 ( #7343, #585, #4427, #7438 ),
 .UNSPECIFIED., .F., .F.,
 ( 4, 4 ),
 ( 0.000000000000000000, 0.001643226871903045875 ),
 .UNSPECIFIED. ) ;
#6332=EDGE_CURVE ( 'NONE', #1017, #3027, #4036, .T. ) ;
#6333=FACE_OUTER_BOUND ( 'NONE', #6233, .T. ) ;
#6334=VECTOR ( 'NONE', #4947, 1000.000000000000114 ) ;
#6336=ORIENTED_EDGE ( 'NONE', *, *, #6425, .F. ) ;
#6337=DIRECTION ( 'NONE',  ( 0.000000000000000000, 1.000000000000000000, 0.000000000000000000 ) ) ;
#6342=DIRECTION ( 'NONE',  ( 0.000000000000000000, 1.000000000000000000, 0.000000000000000000 ) ) ;
#6345=CARTESIAN_POINT ( 'NONE',  ( 28.34870838944214100, 59.99999999999999289, 9.815840903884559765 ) ) ;
#6348=ADVANCED_FACE ( 'NONE', ( #5464 ), #2129, .T. ) ;
#6352=VERTEX_POINT ( 'NONE', #3883 ) ;
#6353=CARTESIAN_POINT ( 'NONE',  ( 33.06426808735054124, 49.99999999999999289, 5.562309845534586294 ) ) ;
#6355=VERTEX_POINT ( 'NONE', #6773 ) ;
#6358=DIRECTION ( 'NONE',  ( 1.000000000000000000, 0.000000000000000000, -0.000000000000000000 ) ) ;
#6361=DIRECTION ( 'NONE',  ( -0.6195972517514877209, 0.000000000000000000, -0.7849198975831889191 ) ) ;
#6369=PLANE ( 'NONE',  #828 ) ;
#6381=AXIS2_PLACEMENT_3D ( 'NONE', #8046, #2894, #7207 ) ;
#6382=CARTESIAN_POINT ( 'NONE',  ( 0.000000000000000000, 30.00000000000000000, 0.000000000000000000 ) ) ;
#6383=AXIS2_PLACEMENT_3D ( 'NONE', #4042, #101, #8487 ) ;
#6386=ORIENTED_EDGE ( 'NONE', *, *, #2862, .T. ) ;
#6388=VECTOR ( 'NONE', #1790, 1000.000000000000000 ) ;
#6390=ORIENTED_EDGE ( 'NONE', *, *, #5695, .F. ) ;
#6392=CARTESIAN_POINT ( 'NONE',  ( 0.000000000000000000, 30.99999999999998579, 0.000000000000000000 ) ) ;
#6397=CIRCLE ( 'NONE', #5144, 30.00000000000000711 ) ;
#6401=ORIENTED_EDGE ( 'NONE', *, *, #5166, .F. ) ;
#6402=DIRECTION ( 'NONE',  ( 0.9449569463147374782, 0.000000000000000000, 0.3271946967961528174 ) ) ;
#6407=DIRECTION ( 'NONE',  ( 0.000000000000000000, 0.000000000000000000, 1.000000000000000000 ) ) ;
#6410=DIRECTION ( 'NONE',  ( 0.000000000000000000, 0.000000000000000000, 1.000000000000000000 ) ) ;
#6412=ORIENTED_EDGE ( 'NONE', *, *, #6485, .T. ) ;
#6413=CARTESIAN_POINT ( 'NONE',  ( 0.000000000000000000, 59.99999999999999289, 0.000000000000000000 ) ) ;
#6415=ORIENTED_EDGE ( 'NONE', *, *, #2987, .F. ) ;
#6420=EDGE_CURVE ( 'NONE', #1992, #3235, #1989, .T. ) ;
#6422=CARTESIAN_POINT ( 'NONE',  ( 4.898587196589413815E-15, 30.99999999999998579, 40.00000000000000711 ) ) ;
#6424=LINE ( 'NONE', #9347, #1668 ) ;
#6425=EDGE_CURVE ( 'NONE', #5052, #7534, #7880, .T. ) ;
#6426=ORIENTED_EDGE ( 'NONE', *, *, #7038, .T. ) ;
#6427=DIRECTION ( 'NONE',  ( -0.000000000000000000, -1.000000000000000000, -0.000000000000000000 ) ) ;
#6430=DIRECTION ( 'NONE',  ( 0.000000000000000000, 1.000000000000000000, 0.000000000000000000 ) ) ;
#6432=VERTEX_POINT ( 'NONE', #9457 ) ;
#6433=CARTESIAN_POINT ( 'NONE',  ( -38.00000000000000711, 59.99999999999999289, -3.980288726281173287E-13 ) ) ;
#6434=DIRECTION ( 'NONE',  ( 0.3286710990610907102, 0.000000000000000000, 0.9444444444444440867 ) ) ;
#6436=DIRECTION ( 'NONE',  ( 0.000000000000000000, 0.7071067811865376918, 0.7071067811865573427 ) ) ;
#6445=ORIENTED_EDGE ( 'NONE', *, *, #106, .T. ) ;
#6449=ADVANCED_FACE ( 'NONE', ( #7778 ), #6696, .T. ) ;
#6451=LINE ( 'NONE', #2798, #1622 ) ;
#6457=VERTEX_POINT ( 'NONE', #7226 ) ;
#6458=AXIS2_PLACEMENT_3D ( 'NONE', #4832, #7847, #1070 ) ;
#6465=CONICAL_SURFACE ( 'NONE', #2197, 26.00000000000000355, 0.7853981633974346233 ) ;
#6467=CARTESIAN_POINT ( 'NONE',  ( -35.48172963891341425, 59.13032414405947179, -4.904055200121582025 ) ) ;
#6469=DIRECTION ( 'NONE',  ( -0.3286710990611142469, 0.000000000000000000, -0.9444444444444359821 ) ) ;
#6470=ORIENTED_EDGE ( 'NONE', *, *, #988, .T. ) ;
#6480=CARTESIAN_POINT ( 'NONE',  ( 29.00000000000000355, 30.00000000000000000, 5.000000000000000888 ) ) ;
#6483=CARTESIAN_POINT ( 'NONE',  ( 4.000000000000001776, 30.00000000000000000, -29.00000000000000355 ) ) ;
#6485=EDGE_CURVE ( 'NONE', #6457, #4542, #1977, .T. ) ;
#6486=PLANE ( 'NONE',  #809 ) ;
#6488=AXIS2_PLACEMENT_3D ( 'NONE', #1334, #2018, #4304 ) ;
#6489=VECTOR ( 'NONE', #3232, 1000.000000000000000 ) ;
#6491=LINE ( 'NONE', #1807, #3389 ) ;
#6497=ORIENTED_EDGE ( 'NONE', *, *, #237, .T. ) ;
#6500=CARTESIAN_POINT ( 'NONE',  ( 10.79742499427301894, 59.99999999999999289, -31.18357922838634977 ) ) ;
#6502=ADVANCED_FACE ( 'NONE', ( #7067 ), #3073, .T. ) ;
#6505=CARTESIAN_POINT ( 'NONE',  ( -23.54759692749571087, 39.99999999999999289, 18.58791755254458877 ) ) ;
#6508=ADVANCED_FACE ( 'NONE', ( #6333 ), #1160, .F. ) ;
#6509=VERTEX_POINT ( 'NONE', #8713 ) ;
#6514=LINE ( 'NONE', #5039, #3494 ) ;
#6517=ORIENTED_EDGE ( 'NONE', *, *, #5138, .F. ) ;
#6525=EDGE_CURVE ( 'NONE', #6748, #8160, #8113, .T. ) ;
#6530=FACE_OUTER_BOUND ( 'NONE', #6919, .T. ) ;
#6532=ORIENTED_EDGE ( 'NONE', *, *, #5585, .T. ) ;
#6533=DIRECTION ( 'NONE',  ( 0.000000000000000000, 0.000000000000000000, -1.000000000000000000 ) ) ;
#6535=DIRECTION ( 'NONE',  ( -1.000000000000000000, 0.000000000000000000, -1.047444401652941269E-14 ) ) ;
#6536=AXIS2_PLACEMENT_3D ( 'NONE', #7987, #3485, #9514 ) ;
#6541=AXIS2_PLACEMENT_3D ( 'NONE', #9200, #6862, #2412 ) ;
#6543=CARTESIAN_POINT ( 'NONE',  ( 4.331874290630489455, 29.33187429063046991, -24.96033808169876878 ) ) ;
#6549=EDGE_CURVE ( 'NONE', #7724, #9229, #3402, .T. ) ;
#6553=LINE ( 'NONE', #8038, #5317 ) ;
#6555=CARTESIAN_POINT ( 'NONE',  ( 5.000000000000002665, 30.00000000000000000, 0.000000000000000000 ) ) ;
#6558=VECTOR ( 'NONE', #6286, 1000.000000000000000 ) ;
#6559=EDGE_CURVE ( 'NONE', #1992, #1652, #7010, .T. ) ;
#6560=DIRECTION ( 'NONE',  ( 0.000000000000000000, 0.000000000000000000, -1.000000000000000000 ) ) ;
#6564=ORIENTED_EDGE ( 'NONE', *, *, #2987, .T. ) ;
#6570=ORIENTED_EDGE ( 'NONE', *, *, #7951, .T. ) ;
#6571=CARTESIAN_POINT ( 'NONE',  ( -34.33638591132956464, 59.77059716828893698, -3.404146005973820888 ) ) ;
#6573=CARTESIAN_POINT ( 'NONE',  ( 35.23154690738756756, 59.33548969180893806, 4.305939634252488268 ) ) ;
#6574=ORIENTED_EDGE ( 'NONE', *, *, #1553, .F. ) ;
#6576=ORIENTED_EDGE ( 'NONE', *, *, #337, .F. ) ;
#6578=DIRECTION ( 'NONE',  ( -0.000000000000000000, -1.000000000000000000, -0.000000000000000000 ) ) ;
#6584=VERTEX_POINT ( 'NONE', #1352 ) ;
#6587=CARTESIAN_POINT ( 'NONE',  ( 0.000000000000000000, 39.99999999999999289, 0.000000000000000000 ) ) ;
#6589=CARTESIAN_POINT ( 'NONE',  ( -4.331874290630493007, 29.33187429063046991, -24.96033808169876878 ) ) ;
#6593=EDGE_LOOP ( 'NONE', ( #1449, #6570, #2567, #7327, #5142 ) ) ;
#6600=ORIENTED_EDGE ( 'NONE', *, *, #2255, .F. ) ;
#6605=LINE ( 'NONE', #5868, #39 ) ;
#6616=CARTESIAN_POINT ( 'NONE',  ( 35.30849208807571671, 59.27954177615072240, 4.448983360113043517 ) ) ;
#6617=ORIENTED_EDGE ( 'NONE', *, *, #8714, .T. ) ;
#6627=EDGE_CURVE ( 'NONE', #8321, #4095, #7269, .T. ) ;
#6630=LINE ( 'NONE', #1504, #5283 ) ;
#6632=CARTESIAN_POINT ( 'NONE',  ( -4.000000000000005329, 28.99999999999997158, -24.67792535850613334 ) ) ;
#6637=AXIS2_PLACEMENT_3D ( 'NONE', #7887, #6342, #6886 ) ;
#6639=DIRECTION ( 'NONE',  ( -1.084202172485503325E-16, 0.000000000000000000, -1.000000000000000000 ) ) ;
#6641=EDGE_CURVE ( 'NONE', #3567, #4855, #2755, .T. ) ;
#6646=CARTESIAN_POINT ( 'NONE',  ( 4.898587196589413815E-15, 39.99999999999999289, 40.00000000000000711 ) ) ;
#6653=ORIENTED_EDGE ( 'NONE', *, *, #6205, .F. ) ;
#6658=CARTESIAN_POINT ( 'NONE',  ( -35.30849208807571671, 59.27954177615072240, -4.448983360113034635 ) ) ;
#6661=CARTESIAN_POINT ( 'NONE',  ( 35.56420151578587507, 58.98289357006406419, 5.732470078048714335 ) ) ;
#6664=CARTESIAN_POINT ( 'NONE',  ( 0.000000000000000000, 59.99999999999999289, 0.000000000000000000 ) ) ;
#6665=EDGE_CURVE ( 'NONE', #504, #6918, #4045, .T. ) ;
#6666=ORIENTED_EDGE ( 'NONE', *, *, #5030, .T. ) ;
#6671=DIRECTION ( 'NONE',  ( 0.5773502691896205130, 0.5773502691896365002, 0.5773502691896204020 ) ) ;
#6672=DIRECTION ( 'NONE',  ( -0.3286710990611015903, 0.000000000000000000, -0.9444444444444403119 ) ) ;
#6673=ORIENTED_EDGE ( 'NONE', *, *, #6152, .T. ) ;
#6675=DIRECTION ( 'NONE',  ( 1.000000000000000000, -0.000000000000000000, 0.000000000000000000 ) ) ;
#6679=CARTESIAN_POINT ( 'NONE',  ( 29.00000000000000355, 0.000000000000000000, -4.000000000000007105 ) ) ;
#6680=ORIENTED_EDGE ( 'NONE', *, *, #3220, .T. ) ;
#6690=CARTESIAN_POINT ( 'NONE',  ( 30.00000000000000711, 30.00000000000000000, -5.000000000000007994 ) ) ;
#6693=CIRCLE ( 'NONE', #4517, 5.000000000000000888 ) ;
#6694=PLANE ( 'NONE',  #5587 ) ;
#6695=AXIS2_PLACEMENT_3D ( 'NONE', #8733, #1956, #4977 ) ;
#6696=TOROIDAL_SURFACE ( 'NONE', #1822, 33.00000000000000711, 5.000000000000000000 ) ;
#6703=CARTESIAN_POINT ( 'NONE',  ( -29.00000000000000355, 28.99999999999997158, 0.000000000000000000 ) ) ;
#6711=CIRCLE ( 'NONE', #7362, 33.00000000000000711 ) ;
#6714=EDGE_LOOP ( 'NONE', ( #1289, #527, #4389, #9266 ) ) ;
#6717=DIRECTION ( 'NONE',  ( 0.000000000000000000, -0.7071067811865500152, -0.7071067811865451302 ) ) ;
#6718=DIRECTION ( 'NONE',  ( 0.000000000000000000, 0.000000000000000000, 1.000000000000000000 ) ) ;
#6720=EDGE_CURVE ( 'NONE', #1969, #9011, #9113, .T. ) ;
#6726=DIRECTION ( 'NONE',  ( -0.000000000000000000, -1.000000000000000000, -0.000000000000000000 ) ) ;
#6729=CARTESIAN_POINT ( 'NONE',  ( -33.06426808735054124, 59.99576382555915899, -3.062309845534580077 ) ) ;
#6735=DIRECTION ( 'NONE',  ( 0.000000000000000000, -0.000000000000000000, 1.000000000000000000 ) ) ;
#6739=ADVANCED_FACE ( 'NONE', ( #8362 ), #8464, .T. ) ;
#6741=CARTESIAN_POINT ( 'NONE',  ( 4.898587196589413815E-15, 37.99999999999996447, 40.00000000000000711 ) ) ;
#6742=EDGE_LOOP ( 'NONE', ( #2307, #4266, #5508, #7566, #3704, #5347, #9048, #7365, #5500, #4673, #227 ) ) ;
#6745=ORIENTED_EDGE ( 'NONE', *, *, #3964, .F. ) ;
#6748=VERTEX_POINT ( 'NONE', #132 ) ;
#6750=EDGE_LOOP ( 'NONE', ( #2459, #316, #3603, #231 ) ) ;
#6751=CARTESIAN_POINT ( 'NONE',  ( -24.67792535850613334, 28.99999999999997158, -3.999999999999997335 ) ) ;
#6753=DIRECTION ( 'NONE',  ( -0.3271946967961539277, 0.000000000000000000, 0.9449569463147370341 ) ) ;
#6755=DIRECTION ( 'NONE',  ( 0.000000000000000000, 1.000000000000000000, 0.000000000000000000 ) ) ;
#6756=ORIENTED_EDGE ( 'NONE', *, *, #4275, .F. ) ;
#6757=LINE ( 'NONE', #3720, #8909 ) ;
#6759=CIRCLE ( 'NONE', #8681, 30.00000000000001066 ) ;
#6762=EDGE_CURVE ( 'NONE', #9346, #1074, #2859, .T. ) ;
#6763=ADVANCED_FACE ( 'NONE', ( #4710 ), #4617, .F. ) ;
#6765=VERTEX_POINT ( 'NONE', #7620 ) ;
#6766=CARTESIAN_POINT ( 'NONE',  ( -8.070750150710590987, 59.89221580632704445, 33.08193339022353285 ) ) ;
#6773=CARTESIAN_POINT ( 'NONE',  ( -29.00000000000000355, 28.99999999999997158, -3.999999999999996447 ) ) ;
#6776=ADVANCED_FACE ( 'NONE', ( #7674 ), #7716, .T. ) ;
#6777=ORIENTED_EDGE ( 'NONE', *, *, #9508, .T. ) ;
#6778=FACE_OUTER_BOUND ( 'NONE', #9054, .T. ) ;
#6782=EDGE_LOOP ( 'NONE', ( #4836, #6849, #3961, #4768 ) ) ;
#6785=EDGE_CURVE ( 'NONE', #4852, #1097, #8178, .T. ) ;
#6790=ORIENTED_EDGE ( 'NONE', *, *, #8570, .T. ) ;
#6796=VERTEX_POINT ( 'NONE', #3013 ) ;
#6801=DIRECTION ( 'NONE',  ( 3.552713678800500929E-15, 0.000000000000000000, 1.000000000000000000 ) ) ;
#6804=EDGE_LOOP ( 'NONE', ( #1439, #4965, #6179, #6386 ) ) ;
#6810=CARTESIAN_POINT ( 'NONE',  ( -24.96033808169876878, 29.33187429063046991, 4.331874290630497448 ) ) ;
#6811=CARTESIAN_POINT ( 'NONE',  ( -4.999999999999998224, 30.00000000000000000, 25.51470164434615029 ) ) ;
#6812=ORIENTED_EDGE ( 'NONE', *, *, #1071, .T. ) ;
#6820=EDGE_LOOP ( 'NONE', ( #7898, #2595, #218, #2726, #5551 ) ) ;
#6823=CIRCLE ( 'NONE', #4317, 37.99999999999999289 ) ;
#6826=ADVANCED_FACE ( 'NONE', ( #7160 ), #6369, .F. ) ;
#6828=DIRECTION ( 'NONE',  ( 0.000000000000000000, -0.000000000000000000, 1.000000000000000000 ) ) ;
#6829=EDGE_LOOP ( 'NONE', ( #2963, #754, #6532, #6653 ) ) ;
#6831=ORIENTED_EDGE ( 'NONE', *, *, #9297, .T. ) ;
#6834=DIRECTION ( 'NONE',  ( 0.5773502691896204020, 0.5773502691896366112, -0.5773502691896204020 ) ) ;
#6838=DIRECTION ( 'NONE',  ( -0.000000000000000000, 1.000000000000000000, -0.000000000000000000 ) ) ;
#6839=DIRECTION ( 'NONE',  ( -0.000000000000000000, -1.000000000000000000, -0.000000000000000000 ) ) ;
#6840=ADVANCED_FACE ( 'NONE', ( #7212 ), #4458, .T. ) ;
#6842=CIRCLE ( 'NONE', #3385, 30.00000000000001066 ) ;
#6843=EDGE_CURVE ( 'NONE', #4855, #3567, #3819, .T. ) ;
#6846=ORIENTED_EDGE ( 'NONE', *, *, #2808, .T. ) ;
#6849=ORIENTED_EDGE ( 'NONE', *, *, #6261, .T. ) ;
#6850=CIRCLE ( 'NONE', #5131, 33.00000000000000711 ) ;
#6851=( GEOMETRIC_REPRESENTATION_CONTEXT ( 3 ) GLOBAL_UNCERTAINTY_ASSIGNED_CONTEXT ( ( #4570 ) ) GLOBAL_UNIT_ASSIGNED_CONTEXT ( ( #2176, #723, #4677 ) ) REPRESENTATION_CONTEXT ( 'NONE', 'WORKASPACE' ) );
#6855=VECTOR ( 'NONE', #59, 1000.000000000000000 ) ;
#6856=AXIS2_PLACEMENT_3D ( 'NONE', #4071, #2622, #2664 ) ;
#6858=CIRCLE ( 'NONE', #8133, 38.00000000000000711 ) ;
#6862=DIRECTION ( 'NONE',  ( 0.7071067811865573427, 0.7071067811865376918, 0.000000000000000000 ) ) ;
#6866=LINE ( 'NONE', #7525, #5590 ) ;
#6869=DIRECTION ( 'NONE',  ( -2.168404344971006649E-16, 0.000000000000000000, -1.000000000000000000 ) ) ;
#6870=DIRECTION ( 'NONE',  ( 0.000000000000000000, 1.000000000000000000, 0.000000000000000000 ) ) ;
#6876=CARTESIAN_POINT ( 'NONE',  ( 4.000000000000002665, 28.99999999999997158, -8.673617379884032514E-16 ) ) ;
#6878=AXIS2_PLACEMENT_3D ( 'NONE', #7900, #595, #7996 ) ;
#6880=ORIENTED_EDGE ( 'NONE', *, *, #6913, .F. ) ;
#6881=LINE ( 'NONE', #8378, #5054 ) ;
#6883=VERTEX_POINT ( 'NONE', #5588 ) ;
#6885=CARTESIAN_POINT ( 'NONE',  ( 7.995545880304246289, 59.98659813632740878, -32.45264704635820152 ) ) ;
#6886=DIRECTION ( 'NONE',  ( 0.000000000000000000, 0.000000000000000000, 1.000000000000000000 ) ) ;
#6888=CARTESIAN_POINT ( 'NONE',  ( -23.54759692749571087, 59.99999999999999289, 18.58791755254458877 ) ) ;
#6893=LINE ( 'NONE', #53, #5422 ) ;
#6895=ORIENTED_EDGE ( 'NONE', *, *, #535, .T. ) ;
#6896=EDGE_CURVE ( 'NONE', #209, #8074, #1835, .T. ) ;
#6897=EDGE_CURVE ( 'NONE', #7710, #8554, #511, .T. ) ;
#6902=CARTESIAN_POINT ( 'NONE',  ( 28.33333333333337833, 59.99999999999999289, -9.860132971832594961 ) ) ;
#6906=ORIENTED_EDGE ( 'NONE', *, *, #1550, .T. ) ;
#6907=CARTESIAN_POINT ( 'NONE',  ( 0.000000000000000000, 30.00000000000000000, 30.00000000000000711 ) ) ;
#6912=ADVANCED_FACE ( 'NONE', ( #1094 ), #9392, .F. ) ;
#6913=EDGE_CURVE ( 'NONE', #8258, #6796, #360, .T. ) ;
#6917=FACE_OUTER_BOUND ( 'NONE', #8801, .T. ) ;
#6918=VERTEX_POINT ( 'NONE', #8508 ) ;
#6919=EDGE_LOOP ( 'NONE', ( #907, #6228, #564, #5198 ) ) ;
#6922=CARTESIAN_POINT ( 'NONE',  ( 38.00000000000000711, 39.99999999999999289, 1.326762908760390927E-13 ) ) ;
#6924=CONICAL_SURFACE ( 'NONE', #2187, 17.99999999999999645, 0.7853981633974447263 ) ;
#6930=CARTESIAN_POINT ( 'NONE',  ( 0.000000000000000000, 59.99999999999999289, 0.000000000000000000 ) ) ;
#6931=CARTESIAN_POINT ( 'NONE',  ( 7.989536001449266678, 59.73029374780621481, -33.69619452719668118 ) ) ;
#6938=CIRCLE ( 'NONE', #5220, 37.99999999999999289 ) ;
#6939=DIRECTION ( 'NONE',  ( 0.3286710990611016459, -0.000000000000000000, 0.9444444444444404230 ) ) ;
#6945=CYLINDRICAL_SURFACE ( 'NONE', #7131, 25.00000000000000000 ) ;
#6946=CARTESIAN_POINT ( 'NONE',  ( 0.000000000000000000, 39.99999999999999289, 0.000000000000000000 ) ) ;
#6953=DIRECTION ( 'NONE',  ( 8.659560562354932858E-17, 0.7071067811865474617, -0.7071067811865474617 ) ) ;
#6954=CARTESIAN_POINT ( 'NONE',  ( 5.000000000000002665, 30.00000000000000000, -29.00000000000000355 ) ) ;
#6959=CIRCLE ( 'NONE', #2214, 38.00000000000000711 ) ;
#6960=EDGE_CURVE ( 'NONE', #6149, #9386, #8603, .T. ) ;
#6962=EDGE_LOOP ( 'NONE', ( #5340, #8862, #8754, #4493 ) ) ;
#6963=CARTESIAN_POINT ( 'NONE',  ( 0.000000000000000000, 39.99999999999999289, -30.00000000000000711 ) ) ;
#6967=ORIENTED_EDGE ( 'NONE', *, *, #7889, .F. ) ;
#6973=ORIENTED_EDGE ( 'NONE', *, *, #1707, .F. ) ;
#6974=CARTESIAN_POINT ( 'NONE',  ( 5.562309845534588959, 59.99999999999999289, -33.06426808735054124 ) ) ;
#6979=VECTOR ( 'NONE', #9370, 1000.000000000000000 ) ;
#6980=DIRECTION ( 'NONE',  ( 0.000000000000000000, 1.000000000000000000, 0.000000000000000000 ) ) ;
#6982=CARTESIAN_POINT ( 'NONE',  ( -33.06426808735054124, 49.99999999999999289, -3.062309845534580077 ) ) ;
#6985=CARTESIAN_POINT ( 'NONE',  ( 5.562309845534588959, 49.99999999999999289, -30.56426808735054479 ) ) ;
#6988=CARTESIAN_POINT ( 'NONE',  ( -10.79742499427301894, 59.99999999999999289, 31.18357922838635332 ) ) ;
#6989=CARTESIAN_POINT ( 'NONE',  ( 5.000000000000009770, 30.00000000000000000, 30.00000000000000711 ) ) ;
#6994=VECTOR ( 'NONE', #448, 1000.000000000000114 ) ;
#6995=DIRECTION ( 'NONE',  ( -0.000000000000000000, -1.000000000000000000, -0.000000000000000000 ) ) ;
#6999=VECTOR ( 'NONE', #9470, 1000.000000000000000 ) ;
#7001=CARTESIAN_POINT ( 'NONE',  ( 30.00000000000000711, 39.99999999999999289, 1.047444401652940259E-13 ) ) ;
#7002=ORIENTED_EDGE ( 'NONE', *, *, #6292, .T. ) ;
#7004=VERTEX_POINT ( 'NONE', #8747 ) ;
#7005=EDGE_CURVE ( 'NONE', #2376, #4857, #3659, .T. ) ;
#7007=EDGE_CURVE ( 'NONE', #8330, #8986, #6514, .T. ) ;
#7008=CYLINDRICAL_SURFACE ( 'NONE', #2124, 25.00000000000000000 ) ;
#7009=AXIS2_PLACEMENT_3D ( 'NONE', #1344, #4369, #8062 ) ;
#7010=CIRCLE ( 'NONE', #9712, 38.00000000000000711 ) ;
#7012=CARTESIAN_POINT ( 'NONE',  ( -35.42756555166880617, 59.00049740791308039, -6.394654627632702315 ) ) ;
#7015=ORIENTED_EDGE ( 'NONE', *, *, #8714, .F. ) ;
#7017=ORIENTED_EDGE ( 'NONE', *, *, #337, .T. ) ;
#7018=ORIENTED_EDGE ( 'NONE', *, *, #4639, .T. ) ;
#7020=VECTOR ( 'NONE', #6082, 1000.000000000000000 ) ;
#7025=EDGE_CURVE ( 'NONE', #7275, #209, #9588, .T. ) ;
#7029=CARTESIAN_POINT ( 'NONE',  ( -3.265277612493196369, 59.85134567364465141, 34.06652594440189574 ) ) ;
#7032=CARTESIAN_POINT ( 'NONE',  ( 5.206952648169308695, 59.04364549838359721, -35.56426808735298550 ) ) ;
#7034=CARTESIAN_POINT ( 'NONE',  ( 0.000000000000000000, 39.99999999999999289, -38.00000000000000711 ) ) ;
#7035=LINE ( 'NONE', #3895, #4914 ) ;
#7038=EDGE_CURVE ( 'NONE', #1527, #6748, #7410, .T. ) ;
#7040=ORIENTED_EDGE ( 'NONE', *, *, #396, .F. ) ;
#7043=ORIENTED_EDGE ( 'NONE', *, *, #2924, .F. ) ;
#7045=DIRECTION ( 'NONE',  ( -1.000000000000000000, 0.000000000000000000, 2.168404344971006649E-16 ) ) ;
#7047=CARTESIAN_POINT ( 'NONE',  ( 0.000000000000000000, 39.99999999999999289, 19.00000000000005684 ) ) ;
#7050=EDGE_LOOP ( 'NONE', ( #1215, #6258 ) ) ;
#7053=CARTESIAN_POINT ( 'NONE',  ( -28.33333333333344939, 59.99999999999999289, 9.860132971832396009 ) ) ;
#7055=EDGE_CURVE ( 'NONE', #4857, #3235, #6959, .T. ) ;
#7056=CARTESIAN_POINT ( 'NONE',  ( -5.562309845534584518, 49.99999999999999289, 33.06426808735054124 ) ) ;
#7057=CARTESIAN_POINT ( 'NONE',  ( -5.562309845534584518, 49.99999999999999289, 33.06426808735054124 ) ) ;
#7060=FACE_OUTER_BOUND ( 'NONE', #9677, .T. ) ;
#7062=EDGE_LOOP ( 'NONE', ( #8158, #2022, #2896, #5493 ) ) ;
#7063=CARTESIAN_POINT ( 'NONE',  ( 34.57348461147494589, 59.39325349372419538, 7.561715963717769107 ) ) ;
#7065=ORIENTED_EDGE ( 'NONE', *, *, #9384, .F. ) ;
#7067=FACE_OUTER_BOUND ( 'NONE', #2462, .T. ) ;
#7068=ADVANCED_FACE ( 'NONE', ( #5090 ), #2854, .T. ) ;
#7070=AXIS2_PLACEMENT_3D ( 'NONE', #9652, #7931, #441 ) ;
#7073=ORIENTED_EDGE ( 'NONE', *, *, #9698, .T. ) ;
#7074=ORIENTED_EDGE ( 'NONE', *, *, #7337, .F. ) ;
#7075=CARTESIAN_POINT ( 'NONE',  ( -24.67792535850613334, 30.00000000000000000, -3.999999999999997335 ) ) ;
#7076=EDGE_CURVE ( 'NONE', #8562, #2569, #5917, .T. ) ;
#7078=CARTESIAN_POINT ( 'NONE',  ( 2.204364238465235033E-15, 38.99999999999993605, -17.99999999999999645 ) ) ;
#7079=DIRECTION ( 'NONE',  ( 0.000000000000000000, 0.000000000000000000, 1.000000000000000000 ) ) ;
#7083=CIRCLE ( 'NONE', #1573, 5.000000000000000888 ) ;
#7084=CIRCLE ( 'NONE', #8360, 4.999999999999997335 ) ;
#7086=EDGE_CURVE ( 'NONE', #4852, #8258, #6605, .T. ) ;
#7088=ORIENTED_EDGE ( 'NONE', *, *, #8815, .F. ) ;
#7089=CARTESIAN_POINT ( 'NONE',  ( 25.51470164434615029, 30.00000000000000000, -5.000000000000007105 ) ) ;
#7099=DIRECTION ( 'NONE',  ( 0.000000000000000000, -0.000000000000000000, 1.000000000000000000 ) ) ;
#7110=CARTESIAN_POINT ( 'NONE',  ( 0.000000000000000000, 39.99999999999999289, -40.00000000000000711 ) ) ;
#7112=DIRECTION ( 'NONE',  ( 0.000000000000000000, 0.000000000000000000, 1.000000000000000000 ) ) ;
#7115=CARTESIAN_POINT ( 'NONE',  ( 0.000000000000000000, 59.99999999999999289, 0.000000000000000000 ) ) ;
#7118=LINE ( 'NONE', #4816, #4353 ) ;
#7119=ORIENTED_EDGE ( 'NONE', *, *, #6186, .F. ) ;
#7123=AXIS2_PLACEMENT_3D ( 'NONE', #7056, #1048, #3457 ) ;
#7128=ORIENTED_EDGE ( 'NONE', *, *, #9110, .T. ) ;
#7129=EDGE_CURVE ( 'NONE', #9400, #5230, #4926, .T. ) ;
#7130=DIRECTION ( 'NONE',  ( -0.000000000000000000, -1.000000000000000000, -0.000000000000000000 ) ) ;
#7131=AXIS2_PLACEMENT_3D ( 'NONE', #207, #6207, #7748 ) ;
#7132=DIRECTION ( 'NONE',  ( -0.000000000000000000, 1.000000000000000000, -0.000000000000000000 ) ) ;
#7135=CARTESIAN_POINT ( 'NONE',  ( 35.90836395996004171, 54.99999999999999289, 12.43339847825378186 ) ) ;
#7138=DIRECTION ( 'NONE',  ( 0.000000000000000000, 0.000000000000000000, 1.000000000000000000 ) ) ;
#7148=LINE ( 'NONE', #8693, #3348 ) ;
#7157=CARTESIAN_POINT ( 'NONE',  ( -31.16666666666624863, 54.99999999999999289, 10.84614626901719170 ) ) ;
#7158=ORIENTED_EDGE ( 'NONE', *, *, #5619, .F. ) ;
#7160=FACE_OUTER_BOUND ( 'NONE', #354, .T. ) ;
#7165=CARTESIAN_POINT ( 'NONE',  ( 33.06426808735054124, 49.99999999999999289, 5.562309845534586294 ) ) ;
#7168=VERTEX_POINT ( 'NONE', #847 ) ;
#7169=CARTESIAN_POINT ( 'NONE',  ( -24.67792535850613334, 30.00000000000000000, 4.000000000000009770 ) ) ;
#7172=CIRCLE ( 'NONE', #7654, 38.00000000000000711 ) ;
#7181=CIRCLE ( 'NONE', #2127, 17.99999999999999645 ) ;
#7184=ORIENTED_EDGE ( 'NONE', *, *, #8731, .T. ) ;
#7188=CARTESIAN_POINT ( 'NONE',  ( 0.000000000000000000, 0.000000000000000000, 29.00000000000000355 ) ) ;
#7192=VECTOR ( 'NONE', #4050, 1000.000000000000000 ) ;
#7193=ORIENTED_EDGE ( 'NONE', *, *, #635, .F. ) ;
#7194=DIRECTION ( 'NONE',  ( 0.5773502691896204020, -0.5773502691896365002, -0.5773502691896205130 ) ) ;
#7200=FACE_OUTER_BOUND ( 'NONE', #7650, .T. ) ;
#7203=ORIENTED_EDGE ( 'NONE', *, *, #1246, .F. ) ;
#7204=DIRECTION ( 'NONE',  ( 0.000000000000000000, -0.000000000000000000, 1.000000000000000000 ) ) ;
#7207=DIRECTION ( 'NONE',  ( 0.000000000000000000, 0.000000000000000000, 1.000000000000000000 ) ) ;
#7209=ADVANCED_FACE ( 'NONE', ( #7656 ), #1582, .F. ) ;
#7212=FACE_OUTER_BOUND ( 'NONE', #3965, .T. ) ;
#7213=CARTESIAN_POINT ( 'NONE',  ( -12.48950176432141923, 59.99999999999999289, -35.88888888888889284 ) ) ;
#7216=ORIENTED_EDGE ( 'NONE', *, *, #6559, .T. ) ;
#7218=EDGE_CURVE ( 'NONE', #5104, #1193, #3992, .T. ) ;
#7219=ORIENTED_EDGE ( 'NONE', *, *, #1001, .F. ) ;
#7221=EDGE_LOOP ( 'NONE', ( #3572, #7128, #3904, #8546, #2952 ) ) ;
#7226=CARTESIAN_POINT ( 'NONE',  ( 5.000000000000008882, 30.00000000000000000, 25.51470164434615029 ) ) ;
#7227=CARTESIAN_POINT ( 'NONE',  ( -24.67792535850613334, 0.000000000000000000, 4.000000000000009770 ) ) ;
#7229=CARTESIAN_POINT ( 'NONE',  ( -4.000000000000005329, 30.00000000000000000, 0.000000000000000000 ) ) ;
#7230=CARTESIAN_POINT ( 'NONE',  ( -3.055999436386194201, 59.99999999999998579, 33.03613408327222345 ) ) ;
#7232=LINE ( 'NONE', #3436, #4092 ) ;
#7242=ORIENTED_EDGE ( 'NONE', *, *, #790, .T. ) ;
#7245=VECTOR ( 'NONE', #3138, 1000.000000000000000 ) ;
#7247=DIRECTION ( 'NONE',  ( -1.000000000000000000, -0.000000000000000000, -3.491481338843134933E-15 ) ) ;
#7249=AXIS2_PLACEMENT_3D ( 'NONE', #674, #9659, #1408 ) ;
#7251=ORIENTED_EDGE ( 'NONE', *, *, #6249, .F. ) ;
#7263=ORIENTED_EDGE ( 'NONE', *, *, #4014, .F. ) ;
#7265=LINE ( 'NONE', #5737, #2918 ) ;
#7269=LINE ( 'NONE', #7321, #4985 ) ;
#7274=ADVANCED_FACE ( 'NONE', ( #9436 ), #8498, .T. ) ;
#7275=VERTEX_POINT ( 'NONE', #397 ) ;
#7288=DIRECTION ( 'NONE',  ( -0.000000000000000000, -1.000000000000000000, -0.000000000000000000 ) ) ;
#7289=ORIENTED_EDGE ( 'NONE', *, *, #1421, .T. ) ;
#7295=CARTESIAN_POINT ( 'NONE',  ( 30.00000000000000711, 59.99999999999999289, 1.047444401652940259E-13 ) ) ;
#7312=DIRECTION ( 'NONE',  ( 0.000000000000000000, 1.000000000000000000, 0.000000000000000000 ) ) ;
#7314=CARTESIAN_POINT ( 'NONE',  ( 35.43299232931641995, 59.17741350630852537, 4.746722514775171042 ) ) ;
#7316=CARTESIAN_POINT ( 'NONE',  ( 12.43339847825378364, 59.99999999999999289, -35.90836395996003461 ) ) ;
#7321=CARTESIAN_POINT ( 'NONE',  ( 23.54759692749571087, 59.99999999999999289, -18.58791755254458167 ) ) ;
#7324=VECTOR ( 'NONE', #1377, 1000.000000000000000 ) ;
#7325=ORIENTED_EDGE ( 'NONE', *, *, #4733, .F. ) ;
#7327=ORIENTED_EDGE ( 'NONE', *, *, #831, .T. ) ;
#7330=EDGE_CURVE ( 'NONE', #137, #4065, #7148, .T. ) ;
#7332=ADVANCED_FACE ( 'NONE', ( #2602 ), #6259, .T. ) ;
#7335=FACE_OUTER_BOUND ( 'NONE', #4890, .T. ) ;
#7337=EDGE_CURVE ( 'NONE', #8061, #7878, #4938, .T. ) ;
#7338=CARTESIAN_POINT ( 'NONE',  ( -3.999999999999998224, 28.99999999999997158, 29.00000000000000355 ) ) ;
#7339=CIRCLE ( 'NONE', #3068, 33.00000000000000711 ) ;
#7340=AXIS2_PLACEMENT_3D ( 'NONE', #9490, #3566, #2861 ) ;
#7343=CARTESIAN_POINT ( 'NONE',  ( 4.000000000000007994, 28.99999999999997158, 24.67792535850613334 ) ) ;
#7344=VERTEX_POINT ( 'NONE', #1083 ) ;
#7347=EDGE_CURVE ( 'NONE', #4501, #4883, #4627, .T. ) ;
#7348=AXIS2_PLACEMENT_3D ( 'NONE', #16, #9108, #5970 ) ;
#7355=VECTOR ( 'NONE', #8109, 1000.000000000000000 ) ;
#7356=ORIENTED_EDGE ( 'NONE', *, *, #4579, .F. ) ;
#7357=CARTESIAN_POINT ( 'NONE',  ( 0.000000000000000000, 59.99999999999999289, 0.000000000000000000 ) ) ;
#7362=AXIS2_PLACEMENT_3D ( 'NONE', #2557, #2611, #6217 ) ;
#7363=DIRECTION ( 'NONE',  ( -0.000000000000000000, -1.000000000000000000, -0.000000000000000000 ) ) ;
#7365=ORIENTED_EDGE ( 'NONE', *, *, #4154, .F. ) ;
#7370=DIRECTION ( 'NONE',  ( -1.000000000000000000, 0.000000000000000000, 2.168404344971006649E-16 ) ) ;
#7372=LINE ( 'NONE', #2120, #6058 ) ;
#7373=EDGE_LOOP ( 'NONE', ( #7946, #8780, #7184, #1285, #8662 ) ) ;
#7375=ORIENTED_EDGE ( 'NONE', *, *, #834, .T. ) ;
#7378=FACE_OUTER_BOUND ( 'NONE', #6782, .T. ) ;
#7379=ORIENTED_EDGE ( 'NONE', *, *, #2924, .T. ) ;
#7380=DIRECTION ( 'NONE',  ( -0.000000000000000000, -1.000000000000000000, -0.000000000000000000 ) ) ;
#7383=LINE ( 'NONE', #531, #5261 ) ;
#7384=CARTESIAN_POINT ( 'NONE',  ( -35.88888888888889284, 59.99999999999999289, 12.48950176432140857 ) ) ;
#7386=DIRECTION ( 'NONE',  ( -0.000000000000000000, -1.000000000000000000, -0.000000000000000000 ) ) ;
#7394=CARTESIAN_POINT ( 'NONE',  ( -29.00000000000000355, 30.00000000000000000, -4.999999999999997335 ) ) ;
#7401=ADVANCED_FACE ( 'NONE', ( #3297 ), #6945, .T. ) ;
#7403=PLANE ( 'NONE',  #2241 ) ;
#7407=CARTESIAN_POINT ( 'NONE',  ( 0.000000000000000000, 59.99999999999999289, 0.000000000000000000 ) ) ;
#7410=LINE ( 'NONE', #2108, #4295 ) ;
#7418=CARTESIAN_POINT ( 'NONE',  ( 0.000000000000000000, 59.99999999999999289, 0.000000000000000000 ) ) ;
#7420=CARTESIAN_POINT ( 'NONE',  ( 34.92646553026882117, 59.22976218012610161, 7.237999934912880740 ) ) ;
#7422=CARTESIAN_POINT ( 'NONE',  ( -5.562309845534584518, 59.99999999999999289, 30.56426808735054124 ) ) ;
#7423=AXIS2_PLACEMENT_3D ( 'NONE', #7229, #5700, #479 ) ;
#7427=CARTESIAN_POINT ( 'NONE',  ( 0.000000000000000000, 39.99999999999999289, -37.99999999999999289 ) ) ;
#7428=VECTOR ( 'NONE', #3875, 1000.000000000000000 ) ;
#7434=CONICAL_SURFACE ( 'NONE', #9173, 37.99999999999999289, 0.7853981633974447263 ) ;
#7436=DIRECTION ( 'NONE',  ( -0.000000000000000000, 1.000000000000000000, -0.000000000000000000 ) ) ;
#7438=CARTESIAN_POINT ( 'NONE',  ( 5.000000000000008882, 30.00000000000000000, 25.51470164434615029 ) ) ;
#7440=DIRECTION ( 'NONE',  ( 0.000000000000000000, 0.000000000000000000, 1.000000000000000000 ) ) ;
#7454=AXIS2_PLACEMENT_3D ( 'NONE', #9239, #7099, #6358 ) ;
#7456=ADVANCED_FACE ( 'NONE', ( #8589 ), #2547, .T. ) ;
#7458=EDGE_CURVE ( 'NONE', #909, #9368, #6451, .T. ) ;
#7463=VECTOR ( 'NONE', #2757, 1000.000000000000000 ) ;
#7467=LINE ( 'NONE', #2552, #2133 ) ;
#7469=CARTESIAN_POINT ( 'NONE',  ( 34.95336322954870667, 59.50565096299369827, 3.917041198934863022 ) ) ;
#7477=DIRECTION ( 'NONE',  ( 0.000000000000000000, -1.000000000000000000, 0.000000000000000000 ) ) ;
#7478=EDGE_LOOP ( 'NONE', ( #9491, #4003, #4025, #2061 ) ) ;
#7486=CYLINDRICAL_SURFACE ( 'NONE', #2667, 38.00000000000000711 ) ;
#7494=AXIS2_PLACEMENT_3D ( 'NONE', #4062, #3359, #4894 ) ;
#7495=VECTOR ( 'NONE', #6839, 1000.000000000000000 ) ;
#7496=CARTESIAN_POINT ( 'NONE',  ( 18.58791755254457811, 59.99999999999999289, 23.54759692749571443 ) ) ;
#7499=AXIS2_PLACEMENT_3D ( 'NONE', #5062, #5112, #5206 ) ;
#7502=VECTOR ( 'NONE', #3574, 1000.000000000000000 ) ;
#7504=DIRECTION ( 'NONE',  ( 0.7071067811865573427, 0.7071067811865376918, 0.000000000000000000 ) ) ;
#7507=ADVANCED_FACE ( 'NONE', ( #7200 ), #1962, .F. ) ;
#7511=DIRECTION ( 'NONE',  ( 0.000000000000000000, 0.000000000000000000, -1.000000000000000000 ) ) ;
#7523=LINE ( 'NONE', #9150, #7834 ) ;
#7525=CARTESIAN_POINT ( 'NONE',  ( 4.653657836759941152E-15, 39.99999999999999289, 37.99999999999999289 ) ) ;
#7527=PLANE ( 'NONE',  #8410 ) ;
#7528=EDGE_CURVE ( 'NONE', #1935, #2408, #2009, .T. ) ;
#7532=CARTESIAN_POINT ( 'NONE',  ( 33.06426808735054124, 59.99576382555915899, 3.062309845534584074 ) ) ;
#7533=ADVANCED_FACE ( 'NONE', ( #5262 ), #4532, .T. ) ;
#7534=VERTEX_POINT ( 'NONE', #6729 ) ;
#7539=DIRECTION ( 'NONE',  ( -0.000000000000000000, -1.000000000000000000, -0.000000000000000000 ) ) ;
#7541=DIRECTION ( 'NONE',  ( -0.9449569463147374782, 0.000000000000000000, -0.3271946967961527619 ) ) ;
#7543=LINE ( 'NONE', #186, #9161 ) ;
#7544=CARTESIAN_POINT ( 'NONE',  ( -5.206952648169303366, 59.04364549838359721, 35.56426808735298550 ) ) ;
#7545=ORIENTED_EDGE ( 'NONE', *, *, #8959, .F. ) ;
#7551=FACE_OUTER_BOUND ( 'NONE', #920, .T. ) ;
#7552=ORIENTED_EDGE ( 'NONE', *, *, #7007, .F. ) ;
#7557=EDGE_LOOP ( 'NONE', ( #410, #2690, #2816, #1151 ) ) ;
#7558=FACE_OUTER_BOUND ( 'NONE', #801, .T. ) ;
#7561=CARTESIAN_POINT ( 'NONE',  ( -30.00000000000001066, 59.99999999999999289, -3.142333204958820777E-13 ) ) ;
#7562=DIRECTION ( 'NONE',  ( -1.000000000000000000, 0.000000000000000000, 0.000000000000000000 ) ) ;
#7566=ORIENTED_EDGE ( 'NONE', *, *, #2945, .F. ) ;
#7568=CARTESIAN_POINT ( 'NONE',  ( -4.665243217607698334, 29.66524321760768501, 25.23917843705063646 ) ) ;
#7570=CARTESIAN_POINT ( 'NONE',  ( 33.06426808735053413, 59.89212256466219486, 8.062309845534588959 ) ) ;
#7574=CARTESIAN_POINT ( 'NONE',  ( 5.562309845534588959, 49.99999999999999289, -33.06426808735054124 ) ) ;
#7584=AXIS2_PLACEMENT_3D ( 'NONE', #5894, #6675, #722 ) ;
#7588=LINE ( 'NONE', #1612, #7728 ) ;
#7589=DIRECTION ( 'NONE',  ( 0.000000000000000000, 0.000000000000000000, 1.000000000000000000 ) ) ;
#7599=DIRECTION ( 'NONE',  ( -0.000000000000000000, -1.000000000000000000, -0.000000000000000000 ) ) ;
#7602=DIRECTION ( 'NONE',  ( 0.7849198975831893632, -0.000000000000000000, -0.6195972517514871658 ) ) ;
#7604=LINE ( 'NONE', #4648, #533 ) ;
#7607=AXIS2_PLACEMENT_3D ( 'NONE', #3362, #312, #1924 ) ;
#7616=VERTEX_POINT ( 'NONE', #6922 ) ;
#7620=CARTESIAN_POINT ( 'NONE',  ( -25.51470164434615029, 30.00000000000000000, -4.999999999999997335 ) ) ;
#7621=VECTOR ( 'NONE', #8211, 1000.000000000000114 ) ;
#7624=EDGE_LOOP ( 'NONE', ( #6445, #1320, #4815, #6574 ) ) ;
#7625=DIRECTION ( 'NONE',  ( 0.3271946967961538166, 0.000000000000000000, -0.9449569463147371451 ) ) ;
#7626=ORIENTED_EDGE ( 'NONE', *, *, #8838, .F. ) ;
#7627=EDGE_LOOP ( 'NONE', ( #5800, #5233, #141, #4011 ) ) ;
#7629=FACE_OUTER_BOUND ( 'NONE', #2930, .T. ) ;
#7632=CARTESIAN_POINT ( 'NONE',  ( 3.070933240276034759, 59.99999999999999289, -32.85680095556730862 ) ) ;
#7633=ADVANCED_FACE ( 'NONE', ( #872 ), #2225, .T. ) ;
#7636=EDGE_CURVE ( 'NONE', #3019, #6432, #9030, .T. ) ;
#7642=ORIENTED_EDGE ( 'NONE', *, *, #4716, .F. ) ;
#7644=VECTOR ( 'NONE', #5028, 1000.000000000000114 ) ;
#7645=VECTOR ( 'NONE', #8237, 999.9999999999998863 ) ;
#7646=ADVANCED_FACE ( 'NONE', ( #7629 ), #5417, .F. ) ;
#7650=EDGE_LOOP ( 'NONE', ( #6315, #6426, #9674, #912 ) ) ;
#7654=AXIS2_PLACEMENT_3D ( 'NONE', #3568, #2162, #9544 ) ;
#7656=FACE_OUTER_BOUND ( 'NONE', #6820, .T. ) ;
#7659=CIRCLE ( 'NONE', #2594, 37.99999999999999289 ) ;
#7665=AXIS2_PLACEMENT_3D ( 'NONE', #1211, #4177, #5697 ) ;
#7670=DIRECTION ( 'NONE',  ( 0.000000000000000000, 1.000000000000000000, -0.000000000000000000 ) ) ;
#7671=ORIENTED_EDGE ( 'NONE', *, *, #7076, .T. ) ;
#7672=CIRCLE ( 'NONE', #8140, 25.00000000000000000 ) ;
#7674=FACE_OUTER_BOUND ( 'NONE', #8752, .T. ) ;
#7685=ORIENTED_EDGE ( 'NONE', *, *, #6762, .T. ) ;
#7686=DIRECTION ( 'NONE',  ( 0.3271946967961527619, 0.000000000000000000, -0.9449569463147374782 ) ) ;
#7687=CARTESIAN_POINT ( 'NONE',  ( 0.000000000000000000, 54.99999999999999289, 0.000000000000000000 ) ) ;
#7689=EDGE_CURVE ( 'NONE', #3235, #2908, #1558, .T. ) ;
#7692=DIRECTION ( 'NONE',  ( 0.000000000000000000, 0.000000000000000000, 1.000000000000000000 ) ) ;
#7698=CARTESIAN_POINT ( 'NONE',  ( -9.860132971832692661, 39.99999999999999289, -28.33333333333334281 ) ) ;
#7699=CARTESIAN_POINT ( 'NONE',  ( 0.000000000000000000, 28.99999999999997158, 0.000000000000000000 ) ) ;
#7700=ORIENTED_EDGE ( 'NONE', *, *, #7704, .F. ) ;
#7703=ORIENTED_EDGE ( 'NONE', *, *, #2865, .F. ) ;
#7704=EDGE_CURVE ( 'NONE', #1193, #3027, #8474, .T. ) ;
#7706=B_SPLINE_CURVE_WITH_KNOTS ( 'NONE', 3,
 ( #3067, #178, #23, #6087, #6766, #8469, #6131, #3728, #9009, #3017, #9163, #6027, #1494, #3168, #8415, #2217, #812, #5254 ),
 .UNSPECIFIED., .F., .F.,
 ( 4, 2, 2, 2, 2, 2, 2, 2, 4 ),
 ( 0.000000000000000000, 0.0006356152723216966244, 0.001271230544643393249, 0.001906845816965089873, 0.002542461089286786498, 0.003178076361608482038, 0.003813691633930177578, 0.004449306906251873119, 0.005084922178573568659 ),
 .UNSPECIFIED. ) ;
#7707=ADVANCED_FACE ( 'NONE', ( #3076 ), #6239, .T. ) ;
#7708=ADVANCED_FACE ( 'NONE', ( #234 ), #9264, .F. ) ;
#7710=VERTEX_POINT ( 'NONE', #7779 ) ;
#7712=CARTESIAN_POINT ( 'NONE',  ( 23.54469556655648077, 54.99999999999999289, 29.82695610816123022 ) ) ;
#7715=VERTEX_POINT ( 'NONE', #9169 ) ;
#7716=PLANE ( 'NONE',  #8079 ) ;
#7719=CARTESIAN_POINT ( 'NONE',  ( -33.06426808735053413, 59.89212256466219486, -8.062309845534585406 ) ) ;
#7721=ORIENTED_EDGE ( 'NONE', *, *, #7528, .F. ) ;
#7724=VERTEX_POINT ( 'NONE', #140 ) ;
#7727=DIRECTION ( 'NONE',  ( 0.000000000000000000, 1.000000000000000000, 0.000000000000000000 ) ) ;
#7728=VECTOR ( 'NONE', #1653, 1000.000000000000000 ) ;
#7733=CARTESIAN_POINT ( 'NONE',  ( -4.000000000000005329, 28.99999999999997158, 0.000000000000000000 ) ) ;
#7734=CARTESIAN_POINT ( 'NONE',  ( 6.957283601945607465, 59.12244502749634734, -35.14908888799237729 ) ) ;
#7736=DIRECTION ( 'NONE',  ( 0.000000000000000000, -0.000000000000000000, 1.000000000000000000 ) ) ;
#7737=CARTESIAN_POINT ( 'NONE',  ( -29.00000000000000355, 30.00000000000000000, -3.999999999999996447 ) ) ;
#7738=VERTEX_POINT ( 'NONE', #8421 ) ;
#7739=AXIS2_PLACEMENT_3D ( 'NONE', #4188, #1222, #4971 ) ;
#7740=LINE ( 'NONE', #1572, #7495 ) ;
#7741=CARTESIAN_POINT ( 'NONE',  ( 20.99999999999999645, 28.99999999999997158, -4.000000000000006217 ) ) ;
#7742=CARTESIAN_POINT ( 'NONE',  ( 31.16666666666653640, 54.99999999999999289, -10.84614626901635503 ) ) ;
#7744=ORIENTED_EDGE ( 'NONE', *, *, #8209, .F. ) ;
#7747=VERTEX_POINT ( 'NONE', #820 ) ;
#7748=DIRECTION ( 'NONE',  ( 0.000000000000000000, 0.000000000000000000, -1.000000000000000000 ) ) ;
#7749=CARTESIAN_POINT ( 'NONE',  ( -38.00000000000000711, 54.99999999999999289, -3.980288726281173287E-13 ) ) ;
#7752=VERTEX_POINT ( 'NONE', #919 ) ;
#7753=DIRECTION ( 'NONE',  ( 0.000000000000000000, 1.000000000000000000, 0.000000000000000000 ) ) ;
#7757=LINE ( 'NONE', #7001, #3064 ) ;
#7762=ORIENTED_EDGE ( 'NONE', *, *, #4204, .T. ) ;
#7765=AXIS2_PLACEMENT_3D ( 'NONE', #3929, #6281, #86 ) ;
#7768=CARTESIAN_POINT ( 'NONE',  ( -35.03233509200964590, 59.17868483491578502, -7.112484670352356986 ) ) ;
#7771=CARTESIAN_POINT ( 'NONE',  ( 34.30759795839968262, 59.50675430643739361, 7.737048950318289542 ) ) ;
#7778=FACE_OUTER_BOUND ( 'NONE', #3111, .T. ) ;
#7779=CARTESIAN_POINT ( 'NONE',  ( -25.90235662024527841, 59.99999999999999289, 20.44670930779905049 ) ) ;
#7781=ORIENTED_EDGE ( 'NONE', *, *, #5070, .T. ) ;
#7787=DIRECTION ( 'NONE',  ( 0.000000000000000000, 1.000000000000000000, 0.000000000000000000 ) ) ;
#7795=CYLINDRICAL_SURFACE ( 'NONE', #3993, 2.500000000000002220 ) ;
#7796=CARTESIAN_POINT ( 'NONE',  ( 0.000000000000000000, 59.99999999999999289, 0.000000000000000000 ) ) ;
#7797=ORIENTED_EDGE ( 'NONE', *, *, #9698, .F. ) ;
#7798=CARTESIAN_POINT ( 'NONE',  ( -18.58791755254457456, 59.99999999999999289, -23.54759692749571443 ) ) ;
#7801=AXIS2_PLACEMENT_3D ( 'NONE', #7699, #6254, #894 ) ;
#7802=CARTESIAN_POINT ( 'NONE',  ( -31.18357922838635687, 59.99999999999999289, -10.79742499427301539 ) ) ;
#7804=FACE_OUTER_BOUND ( 'NONE', #688, .T. ) ;
#7806=VECTOR ( 'NONE', #2397, 1000.000000000000000 ) ;
#7809=FACE_OUTER_BOUND ( 'NONE', #7221, .T. ) ;
#7812=CARTESIAN_POINT ( 'NONE',  ( -9.815840903884557989, 59.99999999999999289, 28.34870838944214455 ) ) ;
#7816=EDGE_CURVE ( 'NONE', #3235, #2792, #1937, .T. ) ;
#7821=CARTESIAN_POINT ( 'NONE',  ( -35.54742948121823787, 59.05243086228237104, -5.228649803729171985 ) ) ;
#7822=ADVANCED_FACE ( 'NONE', ( #8625 ), #1795, .T. ) ;
#7824=VERTEX_POINT ( 'NONE', #4178 ) ;
#7830=DIRECTION ( 'NONE',  ( 0.000000000000000000, 0.000000000000000000, 1.000000000000000000 ) ) ;
#7834=VECTOR ( 'NONE', #3110, 999.9999999999998863 ) ;
#7838=VERTEX_POINT ( 'NONE', #7227 ) ;
#7840=CARTESIAN_POINT ( 'NONE',  ( -3.147661243663441688, 59.92470504718686897, 33.73534932023822108 ) ) ;
#7841=ORIENTED_EDGE ( 'NONE', *, *, #3154, .F. ) ;
#7842=FACE_OUTER_BOUND ( 'NONE', #8223, .T. ) ;
#7843=CYLINDRICAL_SURFACE ( 'NONE', #2927, 38.00000000000000711 ) ;
#7844=VECTOR ( 'NONE', #4708, 1000.000000000000000 ) ;
#7846=DIRECTION ( 'NONE',  ( 0.000000000000000000, 1.000000000000000000, 0.000000000000000000 ) ) ;
#7847=DIRECTION ( 'NONE',  ( -0.000000000000000000, -1.000000000000000000, -0.000000000000000000 ) ) ;
#7852=PLANE ( 'NONE',  #6153 ) ;
#7855=DIRECTION ( 'NONE',  ( -0.000000000000000000, 1.000000000000000000, -0.000000000000000000 ) ) ;
#7856=CARTESIAN_POINT ( 'NONE',  ( -2.094888803305880518E-13, 59.99999999999999289, 30.00000000000000711 ) ) ;
#7859=DIRECTION ( 'NONE',  ( 0.000000000000000000, -0.000000000000000000, 1.000000000000000000 ) ) ;
#7866=CARTESIAN_POINT ( 'NONE',  ( 32.05305536707737701, 59.99999999999999289, 7.848671329280705322 ) ) ;
#7870=DIRECTION ( 'NONE',  ( -0.6195972517514869438, 1.387778780781445281E-15, -0.7849198975831893632 ) ) ;
#7871=ADVANCED_FACE ( 'NONE', ( #5655 ), #1313, .T. ) ;
#7872=ORIENTED_EDGE ( 'NONE', *, *, #7458, .T. ) ;
#7874=ORIENTED_EDGE ( 'NONE', *, *, #9146, .T. ) ;
#7877=DIRECTION ( 'NONE',  ( -0.000000000000000000, -1.000000000000000000, -0.000000000000000000 ) ) ;
#7878=VERTEX_POINT ( 'NONE', #2968 ) ;
#7880=LINE ( 'NONE', #5743, #264 ) ;
#7885=FACE_OUTER_BOUND ( 'NONE', #3502, .T. ) ;
#7886=EDGE_CURVE ( 'NONE', #7275, #4788, #2031, .T. ) ;
#7887=CARTESIAN_POINT ( 'NONE',  ( 0.000000000000000000, 54.99999999999999289, 0.000000000000000000 ) ) ;
#7888=DIRECTION ( 'NONE',  ( 0.000000000000000000, 1.000000000000000000, 0.000000000000000000 ) ) ;
#7889=EDGE_CURVE ( 'NONE', #9639, #6883, #4417, .T. ) ;
#7893=CIRCLE ( 'NONE', #5677, 38.00000000000000711 ) ;
#7898=ORIENTED_EDGE ( 'NONE', *, *, #4375, .F. ) ;
#7899=CYLINDRICAL_SURFACE ( 'NONE', #8092, 2.500000000000002220 ) ;
#7900=CARTESIAN_POINT ( 'NONE',  ( -5.562309845534584518, 59.99999999999999289, 33.06426808735054124 ) ) ;
#7902=LINE ( 'NONE', #9435, #1480 ) ;
#7903=CARTESIAN_POINT ( 'NONE',  ( -1.084202172485504040E-15, 30.00000000000000000, -5.000000000000003553 ) ) ;
#7905=CIRCLE ( 'NONE', #7739, 25.00000000000000000 ) ;
#7906=CARTESIAN_POINT ( 'NONE',  ( 0.000000000000000000, 39.99999999999999289, 0.000000000000000000 ) ) ;
#7910=DIRECTION ( 'NONE',  ( -1.000000000000000000, -0.000000000000000000, -3.491481338843134933E-15 ) ) ;
#7914=CARTESIAN_POINT ( 'NONE',  ( 24.67792535850613334, 0.000000000000000000, -4.000000000000006217 ) ) ;
#7916=DIRECTION ( 'NONE',  ( -0.000000000000000000, -1.000000000000000000, -0.000000000000000000 ) ) ;
#7921=ORIENTED_EDGE ( 'NONE', *, *, #7086, .T. ) ;
#7923=ORIENTED_EDGE ( 'NONE', *, *, #4031, .T. ) ;
#7925=DIRECTION ( 'NONE',  ( 0.000000000000000000, 1.000000000000000000, 0.000000000000000000 ) ) ;
#7930=ORIENTED_EDGE ( 'NONE', *, *, #3414, .T. ) ;
#7931=DIRECTION ( 'NONE',  ( -0.000000000000000000, -1.000000000000000000, -0.000000000000000000 ) ) ;
#7936=LINE ( 'NONE', #5021, #6999 ) ;
#7937=VECTOR ( 'NONE', #8167, 1000.000000000000000 ) ;
#7943=EDGE_CURVE ( 'NONE', #4065, #3142, #1398, .T. ) ;
#7946=ORIENTED_EDGE ( 'NONE', *, *, #6762, .F. ) ;
#7948=DIRECTION ( 'NONE',  ( 0.000000000000000000, 0.000000000000000000, -1.000000000000000000 ) ) ;
#7951=EDGE_CURVE ( 'NONE', #6352, #5598, #2551, .T. ) ;
#7952=ADVANCED_FACE ( 'NONE', ( #7378 ), #8728, .F. ) ;
#7953=CARTESIAN_POINT ( 'NONE',  ( -4.000000000000005329, 28.99999999999997158, -24.67792535850613334 ) ) ;
#7956=LINE ( 'NONE', #4007, #5601 ) ;
#7960=CARTESIAN_POINT ( 'NONE',  ( -25.90235662024524288, 54.99999999999999289, 20.44670930779909668 ) ) ;
#7961=DIRECTION ( 'NONE',  ( -0.000000000000000000, 1.000000000000000000, -0.000000000000000000 ) ) ;
#7967=ORIENTED_EDGE ( 'NONE', *, *, #2832, .F. ) ;
#7973=CIRCLE ( 'NONE', #7494, 30.00000000000000711 ) ;
#7977=AXIS2_PLACEMENT_3D ( 'NONE', #1925, #5000, #2658 ) ;
#7982=ORIENTED_EDGE ( 'NONE', *, *, #8209, .T. ) ;
#7986=CARTESIAN_POINT ( 'NONE',  ( 5.562309845534588959, 49.99999999999999289, -33.06426808735054124 ) ) ;
#7987=CARTESIAN_POINT ( 'NONE',  ( 29.00000000000000355, 30.00000000000000000, -4.000000000000007105 ) ) ;
#7991=ORIENTED_EDGE ( 'NONE', *, *, #950, .F. ) ;
#7995=CARTESIAN_POINT ( 'NONE',  ( 5.421010862427522170E-16, 30.00000000000000000, 5.000000000000004441 ) ) ;
#7996=DIRECTION ( 'NONE',  ( 0.000000000000000000, 0.000000000000000000, 1.000000000000000000 ) ) ;
#8001=VECTOR ( 'NONE', #590, 1000.000000000000000 ) ;
#8008=EDGE_CURVE ( 'NONE', #2208, #3142, #8249, .T. ) ;
#8009=ADVANCED_FACE ( 'NONE', ( #5160 ), #7527, .F. ) ;
#8010=DIRECTION ( 'NONE',  ( 0.000000000000000000, 0.000000000000000000, 1.000000000000000000 ) ) ;
#8011=LINE ( 'NONE', #7213, #3719 ) ;
#8013=EDGE_LOOP ( 'NONE', ( #2216, #4681, #4461, #6967 ) ) ;
#8014=CARTESIAN_POINT ( 'NONE',  ( 0.000000000000000000, 39.99999999999999289, 0.000000000000000000 ) ) ;
#8016=LINE ( 'NONE', #5835, #3546 ) ;
#8017=ORIENTED_EDGE ( 'NONE', *, *, #8788, .T. ) ;
#8023=EDGE_LOOP ( 'NONE', ( #2092, #9002, #489, #4956 ) ) ;
#8026=EDGE_LOOP ( 'NONE', ( #4240, #6973, #3902, #7015 ) ) ;
#8027=ORIENTED_EDGE ( 'NONE', *, *, #8696, .T. ) ;
#8029=CARTESIAN_POINT ( 'NONE',  ( -33.00000000000000711, 54.99999999999999289, -3.456566525454705682E-13 ) ) ;
#8034=DIRECTION ( 'NONE',  ( 0.000000000000000000, 0.000000000000000000, 1.000000000000000000 ) ) ;
#8037=CARTESIAN_POINT ( 'NONE',  ( 5.562309845534588959, 49.99999999999999289, -33.06426808735054124 ) ) ;
#8038=CARTESIAN_POINT ( 'NONE',  ( -4.000000000000005329, 0.000000000000000000, -0.000000000000000000 ) ) ;
#8040=AXIS2_PLACEMENT_3D ( 'NONE', #6248, #1068, #3279 ) ;
#8041=CARTESIAN_POINT ( 'NONE',  ( 2.204364238465235033E-15, 1.000000000000014655, -17.99999999999999645 ) ) ;
#8043=CIRCLE ( 'NONE', #2043, 33.00000000000000711 ) ;
#8044=LINE ( 'NONE', #8695, #7324 ) ;
#8045=ORIENTED_EDGE ( 'NONE', *, *, #9581, .T. ) ;
#8046=CARTESIAN_POINT ( 'NONE',  ( 0.000000000000000000, 59.99999999999999289, 0.000000000000000000 ) ) ;
#8048=EDGE_LOOP ( 'NONE', ( #2984, #6812, #7671, #4407 ) ) ;
#8051=B_SPLINE_CURVE_WITH_KNOTS ( 'NONE', 3,
 ( #3892, #970, #6885, #5373, #4780, #8383, #6931, #191, #8482, #1709, #4685, #8426, #7734, #2392, #4587, #4039, #2529, #6195 ),
 .UNSPECIFIED., .F., .F.,
 ( 4, 2, 2, 2, 2, 2, 2, 2, 4 ),
 ( 0.000000000000000000, 0.0006356152723216952150, 0.001271230544643390430, 0.001906845816965085537, 0.002542461089286780860, 0.003178076361608477268, 0.003813691633930173241, 0.004449306906251869649, 0.005084922178573566057 ),
 .UNSPECIFIED. ) ;
#8052=CARTESIAN_POINT ( 'NONE',  ( 33.06426808735054124, 49.99999999999999289, 8.062309845534588959 ) ) ;
#8054=EDGE_CURVE ( 'NONE', #71, #3464, #2779, .T. ) ;
#8061=VERTEX_POINT ( 'NONE', #5353 ) ;
#8062=DIRECTION ( 'NONE',  ( 0.000000000000000000, 0.000000000000000000, 1.000000000000000000 ) ) ;
#8063=ORIENTED_EDGE ( 'NONE', *, *, #8838, .T. ) ;
#8069=DIRECTION ( 'NONE',  ( -0.3271946967961531505, 0.000000000000000000, 0.9449569463147373671 ) ) ;
#8074=VERTEX_POINT ( 'NONE', #999 ) ;
#8075=FACE_OUTER_BOUND ( 'NONE', #4463, .T. ) ;
#8079=AXIS2_PLACEMENT_3D ( 'NONE', #174, #4663, #6869 ) ;
#8081=AXIS2_PLACEMENT_3D ( 'NONE', #3828, #3980, #3175 ) ;
#8083=EDGE_LOOP ( 'NONE', ( #9557, #3588, #979, #6880 ) ) ;
#8084=CARTESIAN_POINT ( 'NONE',  ( -32.21437568466744494, 59.99999999999997868, -7.920020133197000156 ) ) ;
#8086=ORIENTED_EDGE ( 'NONE', *, *, #6559, .F. ) ;
#8092=AXIS2_PLACEMENT_3D ( 'NONE', #6353, #9373, #5626 ) ;
#8105=CARTESIAN_POINT ( 'NONE',  ( -33.40276010569236576, 59.97308474266854716, -3.079737114311556390 ) ) ;
#8106=EDGE_LOOP ( 'NONE', ( #4134, #9465, #60, #557 ) ) ;
#8107=CARTESIAN_POINT ( 'NONE',  ( 33.89029069002005912, 59.89318186371823316, 3.196943324609357262 ) ) ;
#8109=DIRECTION ( 'NONE',  ( -0.000000000000000000, -1.000000000000000000, -0.000000000000000000 ) ) ;
#8113=LINE ( 'NONE', #8905, #7502 ) ;
#8115=CARTESIAN_POINT ( 'NONE',  ( -4.999999999999999112, 30.00000000000000000, 29.00000000000000355 ) ) ;
#8118=EDGE_CURVE ( 'NONE', #7838, #2244, #9667, .T. ) ;
#8121=DIRECTION ( 'NONE',  ( -0.9444444444444403119, 0.000000000000000000, 0.3286710990611015903 ) ) ;
#8124=CIRCLE ( 'NONE', #5453, 30.00000000000000711 ) ;
#8126=VECTOR ( 'NONE', #6184, 1000.000000000000000 ) ;
#8129=LINE ( 'NONE', #2090, #1189 ) ;
#8130=EDGE_CURVE ( 'NONE', #3288, #9011, #6823, .T. ) ;
#8132=AXIS2_PLACEMENT_3D ( 'NONE', #514, #7312, #3510 ) ;
#8133=AXIS2_PLACEMENT_3D ( 'NONE', #3320, #5550, #4908 ) ;
#8134=AXIS2_PLACEMENT_3D ( 'NONE', #6382, #7925, #9497 ) ;
#8138=FACE_OUTER_BOUND ( 'NONE', #2431, .T. ) ;
#8140=AXIS2_PLACEMENT_3D ( 'NONE', #303, #9332, #5577 ) ;
#8145=VERTEX_POINT ( 'NONE', #5686 ) ;
#8148=ORIENTED_EDGE ( 'NONE', *, *, #5825, .T. ) ;
#8152=AXIS2_PLACEMENT_3D ( 'NONE', #734, #8879, #6639 ) ;
#8153=DIRECTION ( 'NONE',  ( 0.000000000000000000, -0.000000000000000000, 1.000000000000000000 ) ) ;
#8158=ORIENTED_EDGE ( 'NONE', *, *, #6173, .F. ) ;
#8160=VERTEX_POINT ( 'NONE', #2509 ) ;
#8161=CARTESIAN_POINT ( 'NONE',  ( 18.58791755254457811, 39.99999999999999289, 23.54759692749571443 ) ) ;
#8167=DIRECTION ( 'NONE',  ( 1.084202172485503325E-16, 0.000000000000000000, 1.000000000000000000 ) ) ;
#8171=DIRECTION ( 'NONE',  ( 1.000000000000000000, -0.000000000000000000, 6.982962677686269077E-15 ) ) ;
#8172=SHAPE_REPRESENTATION_RELATIONSHIP ( 'NONE' , 'NONE' ,  #551, #6085 ) ;
#8176=CARTESIAN_POINT ( 'NONE',  ( -3.070933240276028542, 59.99999999999999289, 32.85680095556730862 ) ) ;
#8177=EDGE_CURVE ( 'NONE', #71, #8145, #4791, .T. ) ;
#8178=B_SPLINE_CURVE_WITH_KNOTS ( 'NONE', 3,
 ( #2369, #5402, #6171, #953 ),
 .UNSPECIFIED., .F., .F.,
 ( 4, 4 ),
 ( 0.000000000000000000, 0.001643226871903046959 ),
 .UNSPECIFIED. ) ;
#8180=ADVANCED_FACE ( 'NONE', ( #9446 ), #7008, .T. ) ;
#8181=ORIENTED_EDGE ( 'NONE', *, *, #6173, .T. ) ;
#8184=PLANE ( 'NONE',  #4672 ) ;
#8186=DIRECTION ( 'NONE',  ( 0.000000000000000000, 1.000000000000000000, 0.000000000000000000 ) ) ;
#8191=ORIENTED_EDGE ( 'NONE', *, *, #2862, .F. ) ;
#8194=EDGE_LOOP ( 'NONE', ( #6673, #9336, #4311, #654, #5245, #6680, #579 ) ) ;
#8196=AXIS2_PLACEMENT_3D ( 'NONE', #5321, #8329, #8423 ) ;
#8198=ORIENTED_EDGE ( 'NONE', *, *, #5775, .T. ) ;
#8200=ORIENTED_EDGE ( 'NONE', *, *, #5358, .T. ) ;
#8202=ORIENTED_EDGE ( 'NONE', *, *, #7330, .T. ) ;
#8207=EDGE_LOOP ( 'NONE', ( #3308, #1173, #9407, #691 ) ) ;
#8209=EDGE_CURVE ( 'NONE', #3142, #2208, #1037, .T. ) ;
#8211=DIRECTION ( 'NONE',  ( -0.3286710990610907657, 0.000000000000000000, -0.9444444444444440867 ) ) ;
#8212=AXIS2_PLACEMENT_3D ( 'NONE', #4424, #7386, #622 ) ;
#8218=AXIS2_PLACEMENT_3D ( 'NONE', #6147, #7787, #7736 ) ;
#8221=LINE ( 'NONE', #1701, #8126 ) ;
#8222=DIRECTION ( 'NONE',  ( 0.000000000000000000, -1.000000000000000000, 0.000000000000000000 ) ) ;
#8223=EDGE_LOOP ( 'NONE', ( #4736, #7874, #4420, #6167, #5803, #3060 ) ) ;
#8229=CARTESIAN_POINT ( 'NONE',  ( 0.000000000000000000, -50.91168824543140659, 0.000000000000000000 ) ) ;
#8230=PLANE ( 'NONE',  #8152 ) ;
#8234=EDGE_CURVE ( 'NONE', #3142, #3425, #9344, .T. ) ;
#8237=DIRECTION ( 'NONE',  ( 0.5773502691896204020, -0.5773502691896366112, -0.5773502691896204020 ) ) ;
#8243=ORIENTED_EDGE ( 'NONE', *, *, #7816, .T. ) ;
#8244=ADVANCED_FACE ( 'NONE', ( #1049 ), #361, .F. ) ;
#8248=EDGE_CURVE ( 'NONE', #2204, #8074, #8011, .T. ) ;
#8249=CIRCLE ( 'NONE', #9515, 40.00000000000000711 ) ;
#8253=LINE ( 'NONE', #6907, #893 ) ;
#8256=ORIENTED_EDGE ( 'NONE', *, *, #8723, .T. ) ;
#8257=LINE ( 'NONE', #4558, #1205 ) ;
#8258=VERTEX_POINT ( 'NONE', #7914 ) ;
#8261=EDGE_CURVE ( 'NONE', #3567, #7715, #9486, .T. ) ;
#8264=CARTESIAN_POINT ( 'NONE',  ( 0.000000000000000000, 38.99999999999993605, 0.000000000000000000 ) ) ;
#8265=FACE_OUTER_BOUND ( 'NONE', #8048, .T. ) ;
#8271=DIRECTION ( 'NONE',  ( 0.000000000000000000, 1.000000000000000000, -0.000000000000000000 ) ) ;
#8274=DIRECTION ( 'NONE',  ( 0.000000000000000000, 1.000000000000000000, 0.000000000000000000 ) ) ;
#8275=CARTESIAN_POINT ( 'NONE',  ( -5.562309845534584518, 49.99999999999999289, 30.56426808735054124 ) ) ;
#8289=CONICAL_SURFACE ( 'NONE', #726, 17.99999999999999645, 0.7853981633974517207 ) ;
#8295=ORIENTED_EDGE ( 'NONE', *, *, #8118, .F. ) ;
#8296=CARTESIAN_POINT ( 'NONE',  ( -23.54759692749571087, 39.99999999999999289, 18.58791755254458522 ) ) ;
#8302=ORIENTED_EDGE ( 'NONE', *, *, #4510, .T. ) ;
#8307=EDGE_CURVE ( 'NONE', #7878, #6355, #697, .T. ) ;
#8308=VECTOR ( 'NONE', #2052, 1000.000000000000000 ) ;
#8310=EDGE_CURVE ( 'NONE', #742, #294, #7659, .T. ) ;
#8312=CARTESIAN_POINT ( 'NONE',  ( -12.43339847825378719, 39.99999999999999289, 35.90836395996003461 ) ) ;
#8317=DIRECTION ( 'NONE',  ( 0.000000000000000000, 0.000000000000000000, 1.000000000000000000 ) ) ;
#8320=LINE ( 'NONE', #2328, #7428 ) ;
#8321=VERTEX_POINT ( 'NONE', #5091 ) ;
#8322=UNCERTAINTY_MEASURE_WITH_UNIT (LENGTH_MEASURE( 1.000000000000000082E-05 ), #5849, 'distance_accuracy_value', 'NONE');
#8323=ORIENTED_EDGE ( 'NONE', *, *, #5226, .T. ) ;
#8326=DIRECTION ( 'NONE',  ( 0.5773502691896204020, 0.5773502691896363892, 0.5773502691896205130 ) ) ;
#8329=DIRECTION ( 'NONE',  ( -0.000000000000000000, -1.000000000000000000, -0.000000000000000000 ) ) ;
#8330=VERTEX_POINT ( 'NONE', #8052 ) ;
#8332=DIRECTION ( 'NONE',  ( -0.000000000000000000, -1.000000000000000000, -0.000000000000000000 ) ) ;
#8336=CARTESIAN_POINT ( 'NONE',  ( 5.562309845534588959, 59.99999999999999289, -33.06426808735054124 ) ) ;
#8354=FACE_OUTER_BOUND ( 'NONE', #7627, .T. ) ;
#8357=ORIENTED_EDGE ( 'NONE', *, *, #6205, .T. ) ;
#8360=AXIS2_PLACEMENT_3D ( 'NONE', #5314, #8917, #720 ) ;
#8362=FACE_OUTER_BOUND ( 'NONE', #774, .T. ) ;
#8364=EDGE_CURVE ( 'NONE', #5147, #4621, #2284, .T. ) ;
#8369=ORIENTED_EDGE ( 'NONE', *, *, #3189, .F. ) ;
#8374=CARTESIAN_POINT ( 'NONE',  ( 0.000000000000000000, 59.99999999999999289, 0.000000000000000000 ) ) ;
#8377=EDGE_LOOP ( 'NONE', ( #4613, #3931, #9504, #3615 ) ) ;
#8378=CARTESIAN_POINT ( 'NONE',  ( -2.094888803305880518E-13, 59.99999999999999289, 30.00000000000000711 ) ) ;
#8380=CARTESIAN_POINT ( 'NONE',  ( -3.976301758542435394, 59.47750853442943253, 35.00401529666655165 ) ) ;
#8383=CARTESIAN_POINT ( 'NONE',  ( 8.033901996508218346, 59.79149928942062786, -33.49300701350801290 ) ) ;
#8386=ORIENTED_EDGE ( 'NONE', *, *, #4810, .T. ) ;
#8387=CARTESIAN_POINT ( 'NONE',  ( 35.88888888888889284, 59.99999999999999289, -12.48950176432140502 ) ) ;
#8391=DIRECTION ( 'NONE',  ( -0.000000000000000000, -1.000000000000000000, -0.000000000000000000 ) ) ;
#8392=EDGE_LOOP ( 'NONE', ( #8913, #4263, #9212, #2994 ) ) ;
#8399=CARTESIAN_POINT ( 'NONE',  ( 0.000000000000000000, 59.99999999999999289, 0.000000000000000000 ) ) ;
#8410=AXIS2_PLACEMENT_3D ( 'NONE', #759, #3767, #9551 ) ;
#8415=CARTESIAN_POINT ( 'NONE',  ( -6.397328100368723014, 58.99819947112212049, 35.43017184758411986 ) ) ;
#8421=CARTESIAN_POINT ( 'NONE',  ( 20.44670930779903983, 59.99999999999999289, 25.90235662024527841 ) ) ;
#8423=DIRECTION ( 'NONE',  ( 0.000000000000000000, 0.000000000000000000, 1.000000000000000000 ) ) ;
#8424=CARTESIAN_POINT ( 'NONE',  ( -35.88888888888889284, 39.99999999999999289, 12.48950176432140857 ) ) ;
#8426=CARTESIAN_POINT ( 'NONE',  ( 7.123219286842092934, 59.18149658568249549, -35.02766888370167919 ) ) ;
#8428=CARTESIAN_POINT ( 'NONE',  ( 1.084202172485504434E-15, 30.00000000000000000, 5.000000000000005329 ) ) ;
#8432=DIRECTION ( 'NONE',  ( 0.000000000000000000, 0.000000000000000000, 1.000000000000000000 ) ) ;
#8434=CARTESIAN_POINT ( 'NONE',  ( 5.000000000000002665, 30.00000000000000000, -25.51470164434615029 ) ) ;
#8439=LINE ( 'NONE', #8493, #9369 ) ;
#8441=ORIENTED_EDGE ( 'NONE', *, *, #8790, .T. ) ;
#8448=CARTESIAN_POINT ( 'NONE',  ( 0.000000000000000000, 30.00000000000000000, -30.00000000000000711 ) ) ;
#8454=VECTOR ( 'NONE', #2568, 1000.000000000000000 ) ;
#8456=VECTOR ( 'NONE', #9716, 1000.000000000000000 ) ;
#8458=CARTESIAN_POINT ( 'NONE',  ( 33.06426808735054124, 49.99999999999999289, 5.562309845534586294 ) ) ;
#8459=CARTESIAN_POINT ( 'NONE',  ( 4.837354856632047030E-15, 30.00000000000000000, -39.00000000000002132 ) ) ;
#8460=LINE ( 'NONE', #9339, #7844 ) ;
#8464=PLANE ( 'NONE',  #984 ) ;
#8469=CARTESIAN_POINT ( 'NONE',  ( -8.033901996508213017, 59.79149928942061365, 33.49300701350799159 ) ) ;
#8474=LINE ( 'NONE', #4773, #2721 ) ;
#8475=AXIS2_PLACEMENT_3D ( 'NONE', #9662, #2790, #8034 ) ;
#8482=CARTESIAN_POINT ( 'NONE',  ( 7.766845228004612522, 59.52671121465669302, -34.26018231648108525 ) ) ;
#8486=ORIENTED_EDGE ( 'NONE', *, *, #4014, .T. ) ;
#8487=DIRECTION ( 'NONE',  ( -1.776356839400250465E-15, 0.000000000000000000, 1.000000000000000000 ) ) ;
#8493=CARTESIAN_POINT ( 'NONE',  ( 4.000000000000002665, 28.99999999999997158, -8.673617379884032514E-16 ) ) ;
#8497=ORIENTED_EDGE ( 'NONE', *, *, #5087, .F. ) ;
#8498=PLANE ( 'NONE',  #4779 ) ;
#8500=ORIENTED_EDGE ( 'NONE', *, *, #3274, .F. ) ;
#8501=CARTESIAN_POINT ( 'NONE',  ( -5.562309845534584518, 59.99999999999999289, 33.06426808735054124 ) ) ;
#8508=CARTESIAN_POINT ( 'NONE',  ( 9.815840903884561541, 59.99999999999999289, -28.34870838944214100 ) ) ;
#8510=VERTEX_POINT ( 'NONE', #6902 ) ;
#8511=CARTESIAN_POINT ( 'NONE',  ( -34.57348461147494589, 59.39325349372419538, -7.561715963717763778 ) ) ;
#8514=DIRECTION ( 'NONE',  ( 0.000000000000000000, 0.000000000000000000, 1.000000000000000000 ) ) ;
#8522=EDGE_LOOP ( 'NONE', ( #4554, #91 ) ) ;
#8526=DIRECTION ( 'NONE',  ( -0.000000000000000000, 1.000000000000000000, -0.000000000000000000 ) ) ;
#8539=DIRECTION ( 'NONE',  ( -0.000000000000000000, -1.000000000000000000, -0.000000000000000000 ) ) ;
#8541=EDGE_CURVE ( 'NONE', #1776, #5052, #1814, .T. ) ;
#8544=EDGE_CURVE ( 'NONE', #3167, #7710, #7339, .T. ) ;
#8546=ORIENTED_EDGE ( 'NONE', *, *, #7704, .T. ) ;
#8554=VERTEX_POINT ( 'NONE', #4500 ) ;
#8557=EDGE_CURVE ( 'NONE', #156, #1097, #3912, .T. ) ;
#8559=DIRECTION ( 'NONE',  ( 0.000000000000000000, 0.000000000000000000, -1.000000000000000000 ) ) ;
#8561=LINE ( 'NONE', #6963, #4044 ) ;
#8562=VERTEX_POINT ( 'NONE', #3149 ) ;
#8563=LINE ( 'NONE', #2515, #8454 ) ;
#8569=AXIS2_PLACEMENT_3D ( 'NONE', #5179, #5129, #9665 ) ;
#8570=EDGE_CURVE ( 'NONE', #1789, #909, #5439, .T. ) ;
#8574=LINE ( 'NONE', #1801, #1172 ) ;
#8575=DIRECTION ( 'NONE',  ( 0.000000000000000000, 0.000000000000000000, 1.000000000000000000 ) ) ;
#8576=CARTESIAN_POINT ( 'NONE',  ( 0.000000000000000000, 59.99999999999999289, 0.000000000000000000 ) ) ;
#8578=FACE_OUTER_BOUND ( 'NONE', #5549, .T. ) ;
#8588=ADVANCED_FACE ( 'NONE', ( #3953 ), #1195, .T. ) ;
#8589=FACE_OUTER_BOUND ( 'NONE', #1395, .T. ) ;
#8590=AXIS2_PLACEMENT_3D ( 'NONE', #6555, #452, #7859 ) ;
#8591=CONICAL_SURFACE ( 'NONE', #1805, 40.00000000000000711, 0.7853981633974482790 ) ;
#8598=CARTESIAN_POINT ( 'NONE',  ( 23.54469556655648077, 39.99999999999999289, 29.82695610816123022 ) ) ;
#8601=ORIENTED_EDGE ( 'NONE', *, *, #4604, .F. ) ;
#8603=LINE ( 'NONE', #9445, #3985 ) ;
#8605=CIRCLE ( 'NONE', #3878, 30.00000000000000711 ) ;
#8614=EDGE_CURVE ( 'NONE', #4883, #4501, #5777, .T. ) ;
#8617=ORIENTED_EDGE ( 'NONE', *, *, #3530, .T. ) ;
#8625=FACE_OUTER_BOUND ( 'NONE', #5123, .T. ) ;
#8635=CARTESIAN_POINT ( 'NONE',  ( 0.000000000000000000, 39.99999999999999289, 0.000000000000000000 ) ) ;
#8639=ORIENTED_EDGE ( 'NONE', *, *, #3236, .F. ) ;
#8641=LINE ( 'NONE', #5488, #5152 ) ;
#8643=FACE_OUTER_BOUND ( 'NONE', #8026, .T. ) ;
#8645=LINE ( 'NONE', #1867, #6558 ) ;
#8649=CARTESIAN_POINT ( 'NONE',  ( -4.000000000000005329, 30.00000000000000000, -24.67792535850613334 ) ) ;
#8654=CARTESIAN_POINT ( 'NONE',  ( 0.000000000000000000, 30.00000000000000000, 0.000000000000000000 ) ) ;
#8657=ORIENTED_EDGE ( 'NONE', *, *, #5906, .F. ) ;
#8658=DIRECTION ( 'NONE',  ( -0.000000000000000000, -0.000000000000000000, 1.000000000000000000 ) ) ;
#8662=ORIENTED_EDGE ( 'NONE', *, *, #3441, .F. ) ;
#8668=EDGE_CURVE ( 'NONE', #2914, #1527, #3251, .T. ) ;
#8671=CARTESIAN_POINT ( 'NONE',  ( 12.48950176432140680, 39.99999999999999289, 35.88888888888889284 ) ) ;
#8672=ORIENTED_EDGE ( 'NONE', *, *, #6641, .F. ) ;
#8681=AXIS2_PLACEMENT_3D ( 'NONE', #9243, #9381, #2606 ) ;
#8682=EDGE_CURVE ( 'NONE', #8947, #6014, #6397, .T. ) ;
#8684=CARTESIAN_POINT ( 'NONE',  ( 30.00000000000000711, 59.99999999999999289, 1.047444401652940259E-13 ) ) ;
#8686=LINE ( 'NONE', #1909, #6994 ) ;
#8688=VERTEX_POINT ( 'NONE', #7749 ) ;
#8689=CARTESIAN_POINT ( 'NONE',  ( -35.90836395996003461, 54.99999999999999289, -12.43339847825377475 ) ) ;
#8693=CARTESIAN_POINT ( 'NONE',  ( 4.653657836759942730E-15, 59.99999999999999289, -38.00000000000000711 ) ) ;
#8694=CONICAL_SURFACE ( 'NONE', #4274, 40.00000000000000711, 0.7853981633974482790 ) ;
#8695=CARTESIAN_POINT ( 'NONE',  ( -30.00000000000001066, 59.99999999999999289, -3.252551416882082410E-13 ) ) ;
#8696=EDGE_CURVE ( 'NONE', #9233, #1864, #986, .T. ) ;
#8698=VERTEX_POINT ( 'NONE', #7802 ) ;
#8699=CARTESIAN_POINT ( 'NONE',  ( -31.16666666666674601, 59.99999999999999289, 10.84614626901577772 ) ) ;
#8708=CYLINDRICAL_SURFACE ( 'NONE', #9083, 38.00000000000000711 ) ;
#8709=ORIENTED_EDGE ( 'NONE', *, *, #6332, .T. ) ;
#8713=CARTESIAN_POINT ( 'NONE',  ( -33.00000000000000711, 59.99999999999999289, -3.456566525454702653E-13 ) ) ;
#8714=EDGE_CURVE ( 'NONE', #6748, #4852, #7672, .T. ) ;
#8715=AXIS2_PLACEMENT_3D ( 'NONE', #1597, #758, #910 ) ;
#8718=FACE_OUTER_BOUND ( 'NONE', #3863, .T. ) ;
#8719=EDGE_CURVE ( 'NONE', #8510, #1467, #8645, .T. ) ;
#8721=DIRECTION ( 'NONE',  ( 0.000000000000000000, 0.000000000000000000, 1.000000000000000000 ) ) ;
#8723=EDGE_CURVE ( 'NONE', #4855, #8890, #4638, .T. ) ;
#8726=DIRECTION ( 'NONE',  ( 0.000000000000000000, 0.000000000000000000, 1.000000000000000000 ) ) ;
#8727=FACE_OUTER_BOUND ( 'NONE', #5738, .T. ) ;
#8728=CONICAL_SURFACE ( 'NONE', #5256, 17.99999999999999645, 0.7853981633974447263 ) ;
#8730=EDGE_CURVE ( 'NONE', #5165, #9400, #3885, .T. ) ;
#8731=EDGE_CURVE ( 'NONE', #7747, #252, #3930, .T. ) ;
#8732=ORIENTED_EDGE ( 'NONE', *, *, #8130, .T. ) ;
#8733=CARTESIAN_POINT ( 'NONE',  ( -18.58791755254458167, 59.99999999999999289, -23.54759692749571087 ) ) ;
#8735=EDGE_CURVE ( 'NONE', #9259, #7747, #8051, .T. ) ;
#8741=DIRECTION ( 'NONE',  ( -1.000000000000000000, 0.000000000000000000, -0.000000000000000000 ) ) ;
#8746=CIRCLE ( 'NONE', #1804, 38.00000000000000711 ) ;
#8747=CARTESIAN_POINT ( 'NONE',  ( 28.34870838944214100, 39.99999999999999289, 9.815840903884559765 ) ) ;
#8748=CARTESIAN_POINT ( 'NONE',  ( -20.44670930779907891, 54.99999999999999289, -25.90235662024525709 ) ) ;
#8751=VECTOR ( 'NONE', #623, 1000.000000000000114 ) ;
#8752=EDGE_LOOP ( 'NONE', ( #5101, #8791, #6273, #4299 ) ) ;
#8753=FACE_OUTER_BOUND ( 'NONE', #1677, .T. ) ;
#8754=ORIENTED_EDGE ( 'NONE', *, *, #6309, .F. ) ;
#8755=DIRECTION ( 'NONE',  ( -0.000000000000000000, 1.000000000000000000, -0.000000000000000000 ) ) ;
#8760=DIRECTION ( 'NONE',  ( -0.000000000000000000, 1.000000000000000000, -0.000000000000000000 ) ) ;
#8761=CARTESIAN_POINT ( 'NONE',  ( 0.000000000000000000, 39.99999999999999289, 0.000000000000000000 ) ) ;
#8780=ORIENTED_EDGE ( 'NONE', *, *, #2990, .T. ) ;
#8784=CYLINDRICAL_SURFACE ( 'NONE', #2087, 2.499999999999998668 ) ;
#8788=EDGE_CURVE ( 'NONE', #1527, #1789, #3231, .T. ) ;
#8790=EDGE_CURVE ( 'NONE', #8258, #8160, #5309, .T. ) ;
#8791=ORIENTED_EDGE ( 'NONE', *, *, #2486, .T. ) ;
#8793=ORIENTED_EDGE ( 'NONE', *, *, #201, .T. ) ;
#8794=FACE_OUTER_BOUND ( 'NONE', #8805, .T. ) ;
#8798=CARTESIAN_POINT ( 'NONE',  ( 0.000000000000000000, 39.99999999999999289, 0.000000000000000000 ) ) ;
#8801=EDGE_LOOP ( 'NONE', ( #9044, #1611, #3066, #130 ) ) ;
#8805=EDGE_LOOP ( 'NONE', ( #2028, #7043, #6600, #8148 ) ) ;
#8809=CARTESIAN_POINT ( 'NONE',  ( -18.58791755254458167, 59.99999999999999289, -23.54759692749571087 ) ) ;
#8810=ORIENTED_EDGE ( 'NONE', *, *, #8730, .F. ) ;
#8811=CYLINDRICAL_SURFACE ( 'NONE', #7499, 40.00000000000000711 ) ;
#8815=EDGE_CURVE ( 'NONE', #1437, #5863, #381, .T. ) ;
#8816=DIRECTION ( 'NONE',  ( 1.000000000000000000, -0.000000000000000000, 1.047444401652940795E-14 ) ) ;
#8820=CIRCLE ( 'NONE', #7070, 30.00000000000000711 ) ;
#8821=CARTESIAN_POINT ( 'NONE',  ( 2.204364238465235033E-15, 38.99999999999993605, -17.99999999999999645 ) ) ;
#8828=LINE ( 'NONE', #3491, #8308 ) ;
#8830=VECTOR ( 'NONE', #8816, 1000.000000000000000 ) ;
#8836=DIRECTION ( 'NONE',  ( 6.982962677686269866E-15, -0.000000000000000000, -1.000000000000000000 ) ) ;
#8838=EDGE_CURVE ( 'NONE', #279, #3425, #1047, .T. ) ;
#8841=DIRECTION ( 'NONE',  ( 0.000000000000000000, 1.000000000000000000, 0.000000000000000000 ) ) ;
#8847=ORIENTED_EDGE ( 'NONE', *, *, #8668, .T. ) ;
#8848=DIRECTION ( 'NONE',  ( -0.000000000000000000, -1.000000000000000000, -0.000000000000000000 ) ) ;
#8854=CARTESIAN_POINT ( 'NONE',  ( -9.815840903884557989, 59.99999999999999289, 28.34870838944214455 ) ) ;
#8856=ADVANCED_FACE ( 'NONE', ( #9596 ), #7843, .T. ) ;
#8862=ORIENTED_EDGE ( 'NONE', *, *, #6047, .F. ) ;
#8863=DIRECTION ( 'NONE',  ( 0.000000000000000000, 1.000000000000000000, 0.000000000000000000 ) ) ;
#8864=ORIENTED_EDGE ( 'NONE', *, *, #2549, .F. ) ;
#8866=CARTESIAN_POINT ( 'NONE',  ( 0.000000000000000000, 54.99999999999999289, 0.000000000000000000 ) ) ;
#8867=( NAMED_UNIT ( * ) PLANE_ANGLE_UNIT ( ) SI_UNIT ( $, .RADIAN. ) );
#8869=AXIS2_PLACEMENT_3D ( 'NONE', #7960, #460, #9253 ) ;
#8873=CARTESIAN_POINT ( 'NONE',  ( 0.000000000000000000, 59.99999999999999289, 0.000000000000000000 ) ) ;
#8876=DIRECTION ( 'NONE',  ( 0.000000000000000000, 1.000000000000000000, 0.000000000000000000 ) ) ;
#8879=DIRECTION ( 'NONE',  ( -0.7071067811865573427, -0.7071067811865376918, 7.666467083416969298E-17 ) ) ;
#8881=AXIS2_PLACEMENT_3D ( 'NONE', #964, #6136, #6095 ) ;
#8882=CONICAL_SURFACE ( 'NONE', #5252, 26.00000000000000355, 0.7853981633974346233 ) ;
#8885=DIRECTION ( 'NONE',  ( -0.000000000000000000, -1.000000000000000000, -0.000000000000000000 ) ) ;
#8887=CARTESIAN_POINT ( 'NONE',  ( -2.094888803305880518E-13, 39.99999999999999289, 30.00000000000000711 ) ) ;
#8890=VERTEX_POINT ( 'NONE', #7422 ) ;
#8891=DIRECTION ( 'NONE',  ( -0.000000000000000000, -1.000000000000000000, -0.000000000000000000 ) ) ;
#8893=EDGE_LOOP ( 'NONE', ( #6181, #1624, #9260, #5280 ) ) ;
#8899=DIRECTION ( 'NONE',  ( -0.000000000000000000, -1.000000000000000000, -0.000000000000000000 ) ) ;
#8902=AXIS2_PLACEMENT_3D ( 'NONE', #5182, #2348, #4444 ) ;
#8905=CARTESIAN_POINT ( 'NONE',  ( 4.000000000000001776, 30.00000000000000000, -24.67792535850613334 ) ) ;
#8907=ADVANCED_FACE ( 'NONE', ( #7885 ), #5662, .F. ) ;
#8908=EDGE_CURVE ( 'NONE', #6352, #5845, #4314, .T. ) ;
#8909=VECTOR ( 'NONE', #6717, 1000.000000000000114 ) ;
#8913=ORIENTED_EDGE ( 'NONE', *, *, #4642, .T. ) ;
#8915=EDGE_LOOP ( 'NONE', ( #739, #6517, #69, #5409, #3304, #8295, #2578, #7762, #238, #5381, #6777, #8027, #7219, #619, #2730, #1332 ) ) ;
#8917=DIRECTION ( 'NONE',  ( -1.000000000000000000, 0.000000000000000000, -0.000000000000000000 ) ) ;
#8918=CIRCLE ( 'NONE', #4348, 19.00000000000000355 ) ;
#8920=LINE ( 'NONE', #5851, #4666 ) ;
#8922=AXIS2_PLACEMENT_3D ( 'NONE', #4955, #471, #6469 ) ;
#8923=CIRCLE ( 'NONE', #5912, 30.00000000000000711 ) ;
#8924=VECTOR ( 'NONE', #475, 1000.000000000000000 ) ;
#8926=ORIENTED_EDGE ( 'NONE', *, *, #6896, .T. ) ;
#8928=CARTESIAN_POINT ( 'NONE',  ( 0.000000000000000000, 59.99999999999999289, 0.000000000000000000 ) ) ;
#8930=AXIS2_PLACEMENT_3D ( 'NONE', #6946, #208, #7511 ) ;
#8937=EDGE_LOOP ( 'NONE', ( #9570, #1958, #5611, #6401 ) ) ;
#8938=DIRECTION ( 'NONE',  ( 0.000000000000000000, 0.000000000000000000, 1.000000000000000000 ) ) ;
#8944=B_SPLINE_CURVE_WITH_KNOTS ( 'NONE', 3,
 ( #5651, #1054, #1744, #4073, #7771, #7063, #1006, #7420, #1438, #5100, #2717, #2815, #1984, #704, #6661, #9686, #5006, #657, #7314, #6616, #6573, #3714, #7469, #3663, #5929, #2911, #1251, #8107, #565, #8952, #9492, #9638 ),
 .UNSPECIFIED., .F., .F.,
 ( 4, 2, 2, 2, 2, 2, 2, 2, 2, 2, 2, 2, 2, 2, 2, 4 ),
 ( 0.001042552523569530588, 0.002052900844284174554, 0.002558075004641499357, 0.003063249164998824593, 0.003568423325356149395, 0.004073597485713474631, 0.004578771646070799867, 0.005083945806428125103, 0.005589119966785450339, 0.006094294127142775575, 0.006599468287500100810, 0.007104642447857426046, 0.007609816608214751282, 0.008114990768572076518, 0.008620164928929401754, 0.009125339089286726990 ),
 .UNSPECIFIED. ) ;
#8947=VERTEX_POINT ( 'NONE', #3762 ) ;
#8952=CARTESIAN_POINT ( 'NONE',  ( 33.40276010569236576, 59.97308474266854716, 3.079737114311560386 ) ) ;
#8953=VERTEX_POINT ( 'NONE', #6077 ) ;
#8954=CARTESIAN_POINT ( 'NONE',  ( 9.815840903884561541, 39.99999999999999289, -28.34870838944214100 ) ) ;
#8959=EDGE_CURVE ( 'NONE', #909, #2914, #7523, .T. ) ;
#8965=CARTESIAN_POINT ( 'NONE',  ( 0.000000000000000000, 28.99999999999997158, 0.000000000000000000 ) ) ;
#8966=DIRECTION ( 'NONE',  ( 0.000000000000000000, 1.000000000000000000, 0.000000000000000000 ) ) ;
#8971=EDGE_LOOP ( 'NONE', ( #7119, #236, #2801, #9269, #5740, #310 ) ) ;
#8974=LINE ( 'NONE', #5902, #1023 ) ;
#8978=ADVANCED_FACE ( 'NONE', ( #1485 ), #2164, .T. ) ;
#8982=CARTESIAN_POINT ( 'NONE',  ( 0.000000000000000000, 59.99999999999999289, 0.000000000000000000 ) ) ;
#8984=CARTESIAN_POINT ( 'NONE',  ( 5.562309845534588959, 49.99999999999999289, -30.56426808735054479 ) ) ;
#8986=VERTEX_POINT ( 'NONE', #7570 ) ;
#8991=EDGE_CURVE ( 'NONE', #5845, #4065, #3726, .T. ) ;
#8994=VERTEX_POINT ( 'NONE', #8954 ) ;
#9000=FACE_OUTER_BOUND ( 'NONE', #9020, .T. ) ;
#9002=ORIENTED_EDGE ( 'NONE', *, *, #8544, .T. ) ;
#9004=CARTESIAN_POINT ( 'NONE',  ( 33.06426808735054124, 59.99999999999999289, 5.562309845534586294 ) ) ;
#9009=CARTESIAN_POINT ( 'NONE',  ( -7.766845228004613411, 59.52671121465667881, 34.26018231648108525 ) ) ;
#9011=VERTEX_POINT ( 'NONE', #8312 ) ;
#9018=EDGE_CURVE ( 'NONE', #1478, #4857, #8257, .T. ) ;
#9020=EDGE_LOOP ( 'NONE', ( #9117, #4465 ) ) ;
#9028=ORIENTED_EDGE ( 'NONE', *, *, #8541, .F. ) ;
#9030=CIRCLE ( 'NONE', #1303, 39.00000000000002132 ) ;
#9033=EDGE_CURVE ( 'NONE', #9475, #1842, #5475, .T. ) ;
#9039=AXIS2_PLACEMENT_3D ( 'NONE', #8374, #7727, #6828 ) ;
#9040=VECTOR ( 'NONE', #5085, 1000.000000000000000 ) ;
#9044=ORIENTED_EDGE ( 'NONE', *, *, #950, .T. ) ;
#9047=ORIENTED_EDGE ( 'NONE', *, *, #9018, .T. ) ;
#9048=ORIENTED_EDGE ( 'NONE', *, *, #5413, .F. ) ;
#9049=DIRECTION ( 'NONE',  ( -0.000000000000000000, -1.000000000000000000, -0.000000000000000000 ) ) ;
#9050=CARTESIAN_POINT ( 'NONE',  ( -25.51470164434615029, 30.00000000000000000, 5.000000000000010658 ) ) ;
#9051=CARTESIAN_POINT ( 'NONE',  ( -9.815840903884557989, 39.99999999999999289, 28.34870838944214455 ) ) ;
#9054=EDGE_LOOP ( 'NONE', ( #6304, #8045, #8497, #6831, #958 ) ) ;
#9055=DIRECTION ( 'NONE',  ( 8.659560562354904508E-17, -0.7071067811865500152, 0.7071067811865451302 ) ) ;
#9059=VERTEX_POINT ( 'NONE', #908 ) ;
#9061=DIRECTION ( 'NONE',  ( -1.084202172485503448E-16, 0.000000000000000000, -1.000000000000000000 ) ) ;
#9065=DIRECTION ( 'NONE',  ( -6.982962677686274599E-15, 0.000000000000000000, 1.000000000000000000 ) ) ;
#9066=LINE ( 'NONE', #5260, #5274 ) ;
#9067=VECTOR ( 'NONE', #7599, 1000.000000000000000 ) ;
#9072=CARTESIAN_POINT ( 'NONE',  ( -30.00000000000000711, 30.00000000000000000, -4.999999999999997335 ) ) ;
#9074=AXIS2_PLACEMENT_3D ( 'NONE', #4594, #1757, #3090 ) ;
#9083=AXIS2_PLACEMENT_3D ( 'NONE', #7115, #4906, #9402 ) ;
#9094=ADVANCED_FACE ( 'NONE', ( #9000 ), #2209, .T. ) ;
#9095=EDGE_CURVE ( 'NONE', #3425, #279, #736, .T. ) ;
#9098=DIRECTION ( 'NONE',  ( 0.000000000000000000, 1.000000000000000000, 0.000000000000000000 ) ) ;
#9102=EDGE_LOOP ( 'NONE', ( #2811, #6018, #858, #5367 ) ) ;
#9104=AXIS2_PLACEMENT_3D ( 'NONE', #4661, #7670, #4512 ) ;
#9105=CYLINDRICAL_SURFACE ( 'NONE', #3780, 25.00000000000000000 ) ;
#9108=DIRECTION ( 'NONE',  ( 0.000000000000000000, 1.000000000000000000, 0.000000000000000000 ) ) ;
#9110=EDGE_CURVE ( 'NONE', #3204, #3167, #6094, .T. ) ;
#9112=ADVANCED_FACE ( 'NONE', ( #7809 ), #268, .F. ) ;
#9113=LINE ( 'NONE', #1490, #7020 ) ;
#9117=ORIENTED_EDGE ( 'NONE', *, *, #3146, .T. ) ;
#9124=CARTESIAN_POINT ( 'NONE',  ( 24.67792535850613334, 28.99999999999997158, -4.000000000000006217 ) ) ;
#9125=CARTESIAN_POINT ( 'NONE',  ( -3.999999999999999112, 30.00000000000000000, 24.67792535850613334 ) ) ;
#9128=CARTESIAN_POINT ( 'NONE',  ( 5.562309845551833831, 59.00253480853272947, -35.56426808735054834 ) ) ;
#9135=DIRECTION ( 'NONE',  ( 0.6195972517514869438, -1.387778780781445281E-15, 0.7849198975831893632 ) ) ;
#9146=EDGE_CURVE ( 'NONE', #4753, #9229, #6711, .T. ) ;
#9148=CARTESIAN_POINT ( 'NONE',  ( 24.67792535850613334, 28.99999999999997158, 4.000000000000000888 ) ) ;
#9150=CARTESIAN_POINT ( 'NONE',  ( -2.666666666666695384, 27.66666666666662522, -27.66666666666669272 ) ) ;
#9153=VECTOR ( 'NONE', #876, 1000.000000000000227 ) ;
#9154=VECTOR ( 'NONE', #5847, 1000.000000000000000 ) ;
#9155=VECTOR ( 'NONE', #3737, 1000.000000000000000 ) ;
#9161=VECTOR ( 'NONE', #4682, 1000.000000000000000 ) ;
#9163=CARTESIAN_POINT ( 'NONE',  ( -7.420105108763661583, 59.31303094616893645, 34.74949143486232828 ) ) ;
#9165=ORIENTED_EDGE ( 'NONE', *, *, #8908, .T. ) ;
#9169=CARTESIAN_POINT ( 'NONE',  ( -5.562309845551829390, 59.00253480853272947, 35.56426808735054834 ) ) ;
#9170=VERTEX_POINT ( 'NONE', #5541 ) ;
#9171=FACE_OUTER_BOUND ( 'NONE', #6750, .T. ) ;
#9172=CARTESIAN_POINT ( 'NONE',  ( -9.815840903884557989, 59.99999999999999289, 28.34870838944214455 ) ) ;
#9173=AXIS2_PLACEMENT_3D ( 'NONE', #1309, #7477, #1400 ) ;
#9174=CIRCLE ( 'NONE', #5066, 37.99999999999999289 ) ;
#9177=CARTESIAN_POINT ( 'NONE',  ( 3.070933240276034759, 59.99999999999999289, -32.85680095556730862 ) ) ;
#9179=CARTESIAN_POINT ( 'NONE',  ( 29.82695610816121956, 54.99999999999999289, -23.54469556655648077 ) ) ;
#9183=TOROIDAL_SURFACE ( 'NONE', #6637, 33.00000000000000000, 5.000000000000000000 ) ;
#9188=FACE_OUTER_BOUND ( 'NONE', #3477, .T. ) ;
#9192=DIRECTION ( 'NONE',  ( 0.000000000000000000, 1.000000000000000000, 0.000000000000000000 ) ) ;
#9196=AXIS2_PLACEMENT_3D ( 'NONE', #9578, #8274, #1453 ) ;
#9197=ORIENTED_EDGE ( 'NONE', *, *, #1088, .T. ) ;
#9199=CARTESIAN_POINT ( 'NONE',  ( -20.44670930779904339, 59.99999999999999289, -25.90235662024527841 ) ) ;
#9200=CARTESIAN_POINT ( 'NONE',  ( -4.000000000000005329, 28.99999999999997158, 0.000000000000000000 ) ) ;
#9202=DIRECTION ( 'NONE',  ( 0.9444444444444316522, 0.000000000000000000, -0.3286710990611269034 ) ) ;
#9206=AXIS2_PLACEMENT_3D ( 'NONE', #8761, #2673, #1109 ) ;
#9212=ORIENTED_EDGE ( 'NONE', *, *, #1307, .F. ) ;
#9214=ADVANCED_FACE ( 'NONE', ( #1045 ), #1779, .F. ) ;
#9215=EDGE_CURVE ( 'NONE', #5855, #1789, #5448, .T. ) ;
#9216=EDGE_CURVE ( 'NONE', #3216, #6218, #8460, .T. ) ;
#9219=EDGE_LOOP ( 'NONE', ( #9028, #3109, #5400, #6336 ) ) ;
#9220=DIRECTION ( 'NONE',  ( 0.000000000000000000, 0.000000000000000000, 1.000000000000000000 ) ) ;
#9224=CARTESIAN_POINT ( 'NONE',  ( 3.516611797194487465, 59.70849920474193340, -34.51129295977867883 ) ) ;
#9227=AXIS2_PLACEMENT_3D ( 'NONE', #3093, #8391, #8938 ) ;
#9229=VERTEX_POINT ( 'NONE', #5639 ) ;
#9232=DIRECTION ( 'NONE',  ( -0.9444444444444404230, -1.387778780781445281E-15, 0.3286710990611014238 ) ) ;
#9233=VERTEX_POINT ( 'NONE', #9389 ) ;
#9234=CARTESIAN_POINT ( 'NONE',  ( 0.000000000000000000, 30.00000000000000000, 0.000000000000000000 ) ) ;
#9236=VERTEX_POINT ( 'NONE', #948 ) ;
#9239=CARTESIAN_POINT ( 'NONE',  ( 0.000000000000000000, 30.00000000000000000, 29.00000000000000355 ) ) ;
#9242=VECTOR ( 'NONE', #3367, 1000.000000000000000 ) ;
#9243=CARTESIAN_POINT ( 'NONE',  ( 0.000000000000000000, 59.99999999999999289, 0.000000000000000000 ) ) ;
#9245=CIRCLE ( 'NONE', #5773, 2.499999999999998668 ) ;
#9247=FACE_OUTER_BOUND ( 'NONE', #3927, .T. ) ;
#9248=CARTESIAN_POINT ( 'NONE',  ( -25.23917843705063646, 29.66524321760768501, 4.665243217607709880 ) ) ;
#9249=DIRECTION ( 'NONE',  ( -0.000000000000000000, -1.000000000000000000, -0.000000000000000000 ) ) ;
#9250=CARTESIAN_POINT ( 'NONE',  ( 7.848671329280706210, 59.99999999999999289, -32.05305536707737701 ) ) ;
#9253=DIRECTION ( 'NONE',  ( -0.7849198975831886971, -1.387778780781445281E-15, 0.6195972517514877209 ) ) ;
#9255=AXIS2_PLACEMENT_3D ( 'NONE', #4803, #4064, #2413 ) ;
#9256=ORIENTED_EDGE ( 'NONE', *, *, #223, .T. ) ;
#9259=VERTEX_POINT ( 'NONE', #9250 ) ;
#9260=ORIENTED_EDGE ( 'NONE', *, *, #810, .T. ) ;
#9263=EDGE_CURVE ( 'NONE', #880, #5898, #3732, .T. ) ;
#9264=CYLINDRICAL_SURFACE ( 'NONE', #8881, 2.500000000000002220 ) ;
#9266=ORIENTED_EDGE ( 'NONE', *, *, #8118, .T. ) ;
#9269=ORIENTED_EDGE ( 'NONE', *, *, #4744, .T. ) ;
#9270=DIRECTION ( 'NONE',  ( -0.000000000000000000, -1.000000000000000000, -0.000000000000000000 ) ) ;
#9272=CARTESIAN_POINT ( 'NONE',  ( 3.339929591309186652, 59.80724097760847968, -34.22175998453048607 ) ) ;
#9273=DIRECTION ( 'NONE',  ( 8.659560562354962440E-17, 0.7071067811865451302, -0.7071067811865500152 ) ) ;
#9282=ADVANCED_FACE ( 'NONE', ( #9188 ), #5927, .T. ) ;
#9295=ORIENTED_EDGE ( 'NONE', *, *, #5529, .T. ) ;
#9297=EDGE_CURVE ( 'NONE', #6014, #7004, #8641, .T. ) ;
#9300=CARTESIAN_POINT ( 'NONE',  ( -35.54672840350796292, 58.97502204235875922, -5.902312647278756153 ) ) ;
#9301=VERTEX_POINT ( 'NONE', #2402 ) ;
#9302=CARTESIAN_POINT ( 'NONE',  ( -33.06426808735053413, 59.89212256466219486, -8.062309845534585406 ) ) ;
#9303=CIRCLE ( 'NONE', #783, 33.00000000000000711 ) ;
#9304=AXIS2_PLACEMENT_3D ( 'NONE', #8866, #1900, #2784 ) ;
#9308=DIRECTION ( 'NONE',  ( 0.000000000000000000, 0.000000000000000000, 1.000000000000000000 ) ) ;
#9313=CARTESIAN_POINT ( 'NONE',  ( 3.976301758542440279, 59.47750853442942542, -35.00401529666653033 ) ) ;
#9314=CARTESIAN_POINT ( 'NONE',  ( 23.54759692749571443, 59.99999999999999289, -18.58791755254457811 ) ) ;
#9320=CARTESIAN_POINT ( 'NONE',  ( -28.33333333333344939, 59.99999999999999289, 9.860132971832396009 ) ) ;
#9326=ORIENTED_EDGE ( 'NONE', *, *, #4051, .F. ) ;
#9327=LINE ( 'NONE', #7798, #2740 ) ;
#9329=CARTESIAN_POINT ( 'NONE',  ( 0.000000000000000000, 39.99999999999999289, 0.000000000000000000 ) ) ;
#9330=EDGE_CURVE ( 'NONE', #179, #2965, #6204, .T. ) ;
#9332=DIRECTION ( 'NONE',  ( 0.000000000000000000, -1.000000000000000000, 0.000000000000000000 ) ) ;
#9333=CARTESIAN_POINT ( 'NONE',  ( 0.000000000000000000, 1.000000000000014655, 0.000000000000000000 ) ) ;
#9335=DIRECTION ( 'NONE',  ( -1.000000000000000000, 0.000000000000000000, 2.168404344971006649E-16 ) ) ;
#9336=ORIENTED_EDGE ( 'NONE', *, *, #1694, .T. ) ;
#9338=ORIENTED_EDGE ( 'NONE', *, *, #2969, .F. ) ;
#9339=CARTESIAN_POINT ( 'NONE',  ( 0.000000000000000000, 28.99999999999997158, 29.00000000000000355 ) ) ;
#9344=LINE ( 'NONE', #7110, #4349 ) ;
#9346=VERTEX_POINT ( 'NONE', #3248 ) ;
#9347=CARTESIAN_POINT ( 'NONE',  ( 18.58791755254457811, 59.99999999999999289, 23.54759692749571443 ) ) ;
#9350=CARTESIAN_POINT ( 'NONE',  ( 35.90836395996004171, 39.99999999999999289, 12.43339847825378186 ) ) ;
#9351=ORIENTED_EDGE ( 'NONE', *, *, #9263, .F. ) ;
#9355=CARTESIAN_POINT ( 'NONE',  ( 0.000000000000000000, 54.99999999999999289, 0.000000000000000000 ) ) ;
#9358=DIRECTION ( 'NONE',  ( 0.000000000000000000, 0.000000000000000000, 1.000000000000000000 ) ) ;
#9359=EDGE_LOOP ( 'NONE', ( #2290, #9417, #2527, #7379, #9047 ) ) ;
#9365=PLANE ( 'NONE',  #6536 ) ;
#9367=CARTESIAN_POINT ( 'NONE',  ( 29.00000000000000355, 30.00000000000000000, -4.000000000000007105 ) ) ;
#9368=VERTEX_POINT ( 'NONE', #5573 ) ;
#9369=VECTOR ( 'NONE', #4737, 1000.000000000000000 ) ;
#9370=DIRECTION ( 'NONE',  ( -1.000000000000000000, -0.000000000000000000, 1.084202172485503448E-16 ) ) ;
#9371=CARTESIAN_POINT ( 'NONE',  ( -2.094888803305880518E-13, 39.99999999999999289, 30.00000000000000711 ) ) ;
#9373=DIRECTION ( 'NONE',  ( -0.000000000000000000, 1.000000000000000000, -0.000000000000000000 ) ) ;
#9375=ORIENTED_EDGE ( 'NONE', *, *, #1071, .F. ) ;
#9381=DIRECTION ( 'NONE',  ( -0.000000000000000000, -1.000000000000000000, -0.000000000000000000 ) ) ;
#9382=DIRECTION ( 'NONE',  ( 0.000000000000000000, 0.000000000000000000, 1.000000000000000000 ) ) ;
#9384=EDGE_CURVE ( 'NONE', #7724, #5165, #1682, .T. ) ;
#9386=VERTEX_POINT ( 'NONE', #204 ) ;
#9387=CARTESIAN_POINT ( 'NONE',  ( 0.000000000000000000, 59.99999999999999289, -30.00000000000000711 ) ) ;
#9388=ORIENTED_EDGE ( 'NONE', *, *, #4213, .F. ) ;
#9389=CARTESIAN_POINT ( 'NONE',  ( -4.000000000000005329, 0.000000000000000000, -29.00000000000000355 ) ) ;
#9392=PLANE ( 'NONE',  #206 ) ;
#9394=AXIS2_PLACEMENT_3D ( 'NONE', #3610, #5833, #7370 ) ;
#9396=CIRCLE ( 'NONE', #6070, 19.00000000000000355 ) ;
#9400=VERTEX_POINT ( 'NONE', #1030 ) ;
#9402=DIRECTION ( 'NONE',  ( 0.000000000000000000, 0.000000000000000000, -1.000000000000000000 ) ) ;
#9403=EDGE_CURVE ( 'NONE', #1842, #6584, #3997, .T. ) ;
#9404=AXIS2_PLACEMENT_3D ( 'NONE', #6392, #2580, #8575 ) ;
#9406=CARTESIAN_POINT ( 'NONE',  ( 0.000000000000000000, 0.000000000000000000, 0.000000000000000000 ) ) ;
#9407=ORIENTED_EDGE ( 'NONE', *, *, #1548, .T. ) ;
#9409=VERTEX_POINT ( 'NONE', #343 ) ;
#9415=ORIENTED_EDGE ( 'NONE', *, *, #4496, .T. ) ;
#9417=ORIENTED_EDGE ( 'NONE', *, *, #5947, .T. ) ;
#9418=CARTESIAN_POINT ( 'NONE',  ( -9.860132971832692661, 59.99999999999999289, -28.33333333333334281 ) ) ;
#9419=VERTEX_POINT ( 'NONE', #6989 ) ;
#9420=CARTESIAN_POINT ( 'NONE',  ( -32.85680095556730862, 59.99999999999999289, -3.070933240276025877 ) ) ;
#9429=LINE ( 'NONE', #4734, #6979 ) ;
#9431=ORIENTED_EDGE ( 'NONE', *, *, #6549, .T. ) ;
#9435=CARTESIAN_POINT ( 'NONE',  ( 0.000000000000000000, 59.99999999999999289, -30.00000000000000711 ) ) ;
#9436=FACE_OUTER_BOUND ( 'NONE', #9102, .T. ) ;
#9440=LINE ( 'NONE', #2653, #2587 ) ;
#9445=CARTESIAN_POINT ( 'NONE',  ( 33.06426808735054124, 49.99999999999999289, 3.062309845534584074 ) ) ;
#9446=FACE_OUTER_BOUND ( 'NONE', #9489, .T. ) ;
#9454=PLANE ( 'NONE',  #5137 ) ;
#9457=CARTESIAN_POINT ( 'NONE',  ( 0.000000000000000000, 30.00000000000000000, 39.00000000000002132 ) ) ;
#9461=EDGE_CURVE ( 'NONE', #5230, #2792, #4936, .T. ) ;
#9465=ORIENTED_EDGE ( 'NONE', *, *, #4430, .F. ) ;
#9470=DIRECTION ( 'NONE',  ( 0.000000000000000000, 0.000000000000000000, 1.000000000000000000 ) ) ;
#9471=B_SPLINE_CURVE_WITH_KNOTS ( 'NONE', 3,
 ( #7719, #1152, #228, #2469, #5505, #8511, #1742, #4764, #7768, #1003, #1787, #7012, #276, #9300, #2513, #4813, #7821, #6467, #1389, #6658, #9683, #2909, #5926, #9593, #5098, #6571, #563, #1981, #5791, #8105, #5151, #5004 ),
 .UNSPECIFIED., .F., .F.,
 ( 4, 2, 2, 2, 2, 2, 2, 2, 2, 2, 2, 2, 2, 2, 2, 4 ),
 ( 0.001042552523569530588, 0.002052900844284173687, 0.002558075004641498489, 0.003063249164998823292, 0.003568423325356147660, 0.004073597485713472896, 0.004578771646070796397, 0.005083945806428121633, 0.005589119966785446869, 0.006094294127142772105, 0.006599468287500097341, 0.007104642447857422577, 0.007609816608214747813, 0.008114990768572073049, 0.008620164928929398285, 0.009125339089286721786 ),
 .UNSPECIFIED. ) ;
#9475=VERTEX_POINT ( 'NONE', #1960 ) ;
#9480=DIRECTION ( 'NONE',  ( -0.000000000000000000, 1.000000000000000000, -0.000000000000000000 ) ) ;
#9486=LINE ( 'NONE', #313, #725 ) ;
#9489=EDGE_LOOP ( 'NONE', ( #1721, #5649, #8793, #5293 ) ) ;
#9490=CARTESIAN_POINT ( 'NONE',  ( 0.000000000000000000, 59.99999999999999289, 0.000000000000000000 ) ) ;
#9491=ORIENTED_EDGE ( 'NONE', *, *, #2991, .T. ) ;
#9492=CARTESIAN_POINT ( 'NONE',  ( 33.23540996127940872, 59.98874451312625666, 3.062309845534584074 ) ) ;
#9494=ORIENTED_EDGE ( 'NONE', *, *, #1722, .T. ) ;
#9495=EDGE_CURVE ( 'NONE', #2517, #9574, #8828, .T. ) ;
#9497=DIRECTION ( 'NONE',  ( 0.000000000000000000, 0.000000000000000000, 1.000000000000000000 ) ) ;
#9498=VECTOR ( 'NONE', #558, 1000.000000000000000 ) ;
#9500=ORIENTED_EDGE ( 'NONE', *, *, #4510, .F. ) ;
#9501=ORIENTED_EDGE ( 'NONE', *, *, #3291, .F. ) ;
#9503=EDGE_LOOP ( 'NONE', ( #9197, #7074, #5971, #7263 ) ) ;
#9504=ORIENTED_EDGE ( 'NONE', *, *, #8054, .T. ) ;
#9508=EDGE_CURVE ( 'NONE', #9475, #9233, #6553, .T. ) ;
#9512=LINE ( 'NONE', #7188, #5684 ) ;
#9514=DIRECTION ( 'NONE',  ( 0.000000000000000000, 0.000000000000000000, -1.000000000000000000 ) ) ;
#9515=AXIS2_PLACEMENT_3D ( 'NONE', #2131, #2213, #2080 ) ;
#9516=B_SPLINE_CURVE_WITH_KNOTS ( 'NONE', 3,
 ( #6811, #7568, #165, #68 ),
 .UNSPECIFIED., .F., .F.,
 ( 4, 4 ),
 ( 0.000000000000000000, 0.001643226871903046308 ),
 .UNSPECIFIED. ) ;
#9518=CARTESIAN_POINT ( 'NONE',  ( -32.89361530837994962, 59.92713194881500982, -8.062309845534583630 ) ) ;
#9519=CARTESIAN_POINT ( 'NONE',  ( 9.860132971832495485, 59.99999999999999289, 28.33333333333341031 ) ) ;
#9520=EDGE_CURVE ( 'NONE', #4557, #8890, #1367, .T. ) ;
#9525=DIRECTION ( 'NONE',  ( 0.000000000000000000, 0.000000000000000000, 1.000000000000000000 ) ) ;
#9527=FACE_OUTER_BOUND ( 'NONE', #6593, .T. ) ;
#9532=EDGE_LOOP ( 'NONE', ( #5014, #4429, #4535, #2326 ) ) ;
#9536=DIRECTION ( 'NONE',  ( 0.000000000000000000, 0.000000000000000000, 1.000000000000000000 ) ) ;
#9540=CIRCLE ( 'NONE', #1492, 5.000000000000001776 ) ;
#9541=EDGE_LOOP ( 'NONE', ( #308, #6666, #4343, #885 ) ) ;
#9544=DIRECTION ( 'NONE',  ( 0.000000000000000000, 0.000000000000000000, 1.000000000000000000 ) ) ;
#9549=CARTESIAN_POINT ( 'NONE',  ( 0.000000000000000000, 59.99999999999999289, 0.000000000000000000 ) ) ;
#9550=AXIS2_PLACEMENT_3D ( 'NONE', #2428, #819, #2475 ) ;
#9551=DIRECTION ( 'NONE',  ( 0.7849198975831888081, 0.000000000000000000, -0.6195972517514876099 ) ) ;
#9557=ORIENTED_EDGE ( 'NONE', *, *, #7086, .F. ) ;
#9558=CYLINDRICAL_SURFACE ( 'NONE', #3286, 38.00000000000000000 ) ;
#9563=DIRECTION ( 'NONE',  ( -0.6195972517514876099, 0.000000000000000000, -0.7849198975831889191 ) ) ;
#9568=LINE ( 'NONE', #6679, #9155 ) ;
#9569=AXIS2_PLACEMENT_3D ( 'NONE', #7157, #1143, #4164 ) ;
#9570=ORIENTED_EDGE ( 'NONE', *, *, #5945, .F. ) ;
#9571=FACE_OUTER_BOUND ( 'NONE', #6714, .T. ) ;
#9574=VERTEX_POINT ( 'NONE', #5904 ) ;
#9578=CARTESIAN_POINT ( 'NONE',  ( -5.562309845534584518, 49.99999999999999289, 33.06426808735054124 ) ) ;
#9580=ADVANCED_FACE ( 'NONE', ( #5269 ), #8230, .T. ) ;
#9581=EDGE_CURVE ( 'NONE', #5230, #4753, #4377, .T. ) ;
#9588=LINE ( 'NONE', #602, #9498 ) ;
#9592=ORIENTED_EDGE ( 'NONE', *, *, #4770, .T. ) ;
#9593=CARTESIAN_POINT ( 'NONE',  ( -34.72826512091049267, 59.61718548957851027, -3.689690490709783166 ) ) ;
#9596=FACE_OUTER_BOUND ( 'NONE', #7557, .T. ) ;
#9597=EDGE_LOOP ( 'NONE', ( #568, #5377 ) ) ;
#9608=DIRECTION ( 'NONE',  ( 0.000000000000000000, 0.000000000000000000, 1.000000000000000000 ) ) ;
#9636=DIRECTION ( 'NONE',  ( 0.000000000000000000, 1.000000000000000000, 0.000000000000000000 ) ) ;
#9638=CARTESIAN_POINT ( 'NONE',  ( 33.06426808735054124, 59.99576382555915899, 3.062309845534584074 ) ) ;
#9639=VERTEX_POINT ( 'NONE', #4484 ) ;
#9644=AXIS2_PLACEMENT_3D ( 'NONE', #6930, #5559, #190 ) ;
#9648=CIRCLE ( 'NONE', #977, 38.00000000000000000 ) ;
#9650=CARTESIAN_POINT ( 'NONE',  ( -5.666666666666482222, 19.33333333333320780, 19.33333333333351334 ) ) ;
#9652=CARTESIAN_POINT ( 'NONE',  ( 0.000000000000000000, 39.99999999999999289, 0.000000000000000000 ) ) ;
#9654=CARTESIAN_POINT ( 'NONE',  ( 0.000000000000000000, 0.000000000000000000, 0.000000000000000000 ) ) ;
#9659=DIRECTION ( 'NONE',  ( -0.000000000000000000, -1.000000000000000000, -0.000000000000000000 ) ) ;
#9660=ORIENTED_EDGE ( 'NONE', *, *, #4328, .T. ) ;
#9662=CARTESIAN_POINT ( 'NONE',  ( 0.000000000000000000, 38.99999999999993605, 0.000000000000000000 ) ) ;
#9665=DIRECTION ( 'NONE',  ( -0.9449569463147374782, 0.000000000000000000, -0.3271946967961528729 ) ) ;
#9667=CIRCLE ( 'NONE', #61, 25.00000000000000000 ) ;
#9670=DIRECTION ( 'NONE',  ( 0.000000000000000000, 0.000000000000000000, 1.000000000000000000 ) ) ;
#9674=ORIENTED_EDGE ( 'NONE', *, *, #6525, .T. ) ;
#9677=EDGE_LOOP ( 'NONE', ( #6111, #5489, #3805, #8323 ) ) ;
#9683=CARTESIAN_POINT ( 'NONE',  ( -35.23154690738756756, 59.33548969180893806, -4.305939634252483827 ) ) ;
#9684=ADVANCED_FACE ( 'NONE', ( #5477 ), #1618, .T. ) ;
#9686=CARTESIAN_POINT ( 'NONE',  ( 35.56433427405016090, 59.02194934605864063, 5.394111410765026093 ) ) ;
#9687=VERTEX_POINT ( 'NONE', #9179 ) ;
#9688=DIRECTION ( 'NONE',  ( -0.000000000000000000, -1.000000000000000000, -0.000000000000000000 ) ) ;
#9690=CIRCLE ( 'NONE', #7801, 25.00000000000000000 ) ;
#9691=ORIENTED_EDGE ( 'NONE', *, *, #2372, .F. ) ;
#9694=CARTESIAN_POINT ( 'NONE',  ( 0.000000000000000000, 54.99999999999999289, 0.000000000000000000 ) ) ;
#9695=TOROIDAL_SURFACE ( 'NONE', #3211, 33.00000000000000711, 5.000000000000000000 ) ;
#9697=AXIS2_PLACEMENT_3D ( 'NONE', #3551, #6560, #8741 ) ;
#9698=EDGE_CURVE ( 'NONE', #7616, #3887, #9174, .T. ) ;
#9699=ORIENTED_EDGE ( 'NONE', *, *, #2945, .T. ) ;
#9701=EDGE_CURVE ( 'NONE', #3761, #2408, #7035, .T. ) ;
#9703=VECTOR ( 'NONE', #4944, 1000.000000000000000 ) ;
#9705=CARTESIAN_POINT ( 'NONE',  ( -29.00000000000000355, 0.000000000000000000, 4.000000000000010658 ) ) ;
#9707=CARTESIAN_POINT ( 'NONE',  ( 0.000000000000000000, 30.00000000000000000, 0.000000000000000000 ) ) ;
#9709=CIRCLE ( 'NONE', #4351, 33.00000000000000711 ) ;
#9712=AXIS2_PLACEMENT_3D ( 'NONE', #5839, #2030, #5884 ) ;
#9715=DIRECTION ( 'NONE',  ( 0.000000000000000000, 0.000000000000000000, 1.000000000000000000 ) ) ;
#9716=DIRECTION ( 'NONE',  ( -0.000000000000000000, 1.000000000000000000, -0.000000000000000000 ) ) ;
#9717=CARTESIAN_POINT ( 'NONE',  ( 0.000000000000000000, 1.000000000000014655, 0.000000000000000000 ) ) ;
#9718=B_SPLINE_CURVE_WITH_KNOTS ( 'NONE', 3,
 ( #7532, #764, #2375, #864 ),
 .UNSPECIFIED., .F., .F.,
 ( 4, 4 ),
 ( 0.009125339089286726990, 0.009329711147074801203 ),
 .UNSPECIFIED. ) ;
#9736=ADVANCED_FACE ( 'NONE', ( #4186, #7335 ), #6486, .T. ) ;
#9739=CARTESIAN_POINT ( 'NONE',  ( 5.562309845534588959, 49.99999999999999289, -35.56426808735054834 ) ) ;
#9749=EDGE_LOOP ( 'NONE', ( #716, #3550, #8181, #5930, #5046 ) ) ;
#9765=COLOUR_RGB('Dark Blue',0.08,0.2,0.34);
#9766=FILL_AREA_STYLE_COLOUR('',#9765);
#9767=FILL_AREA_STYLE('',(#9766));
#9768=SURFACE_STYLE_FILL_AREA(#9767);
#9769=SURFACE_SIDE_STYLE('',(#9768));
#9770=SURFACE_STYLE_USAGE(.BOTH.,#9769);
#9771=PRESENTATION_STYLE_ASSIGNMENT((#9770));
ENDSEC;
END-ISO-10303-21;
